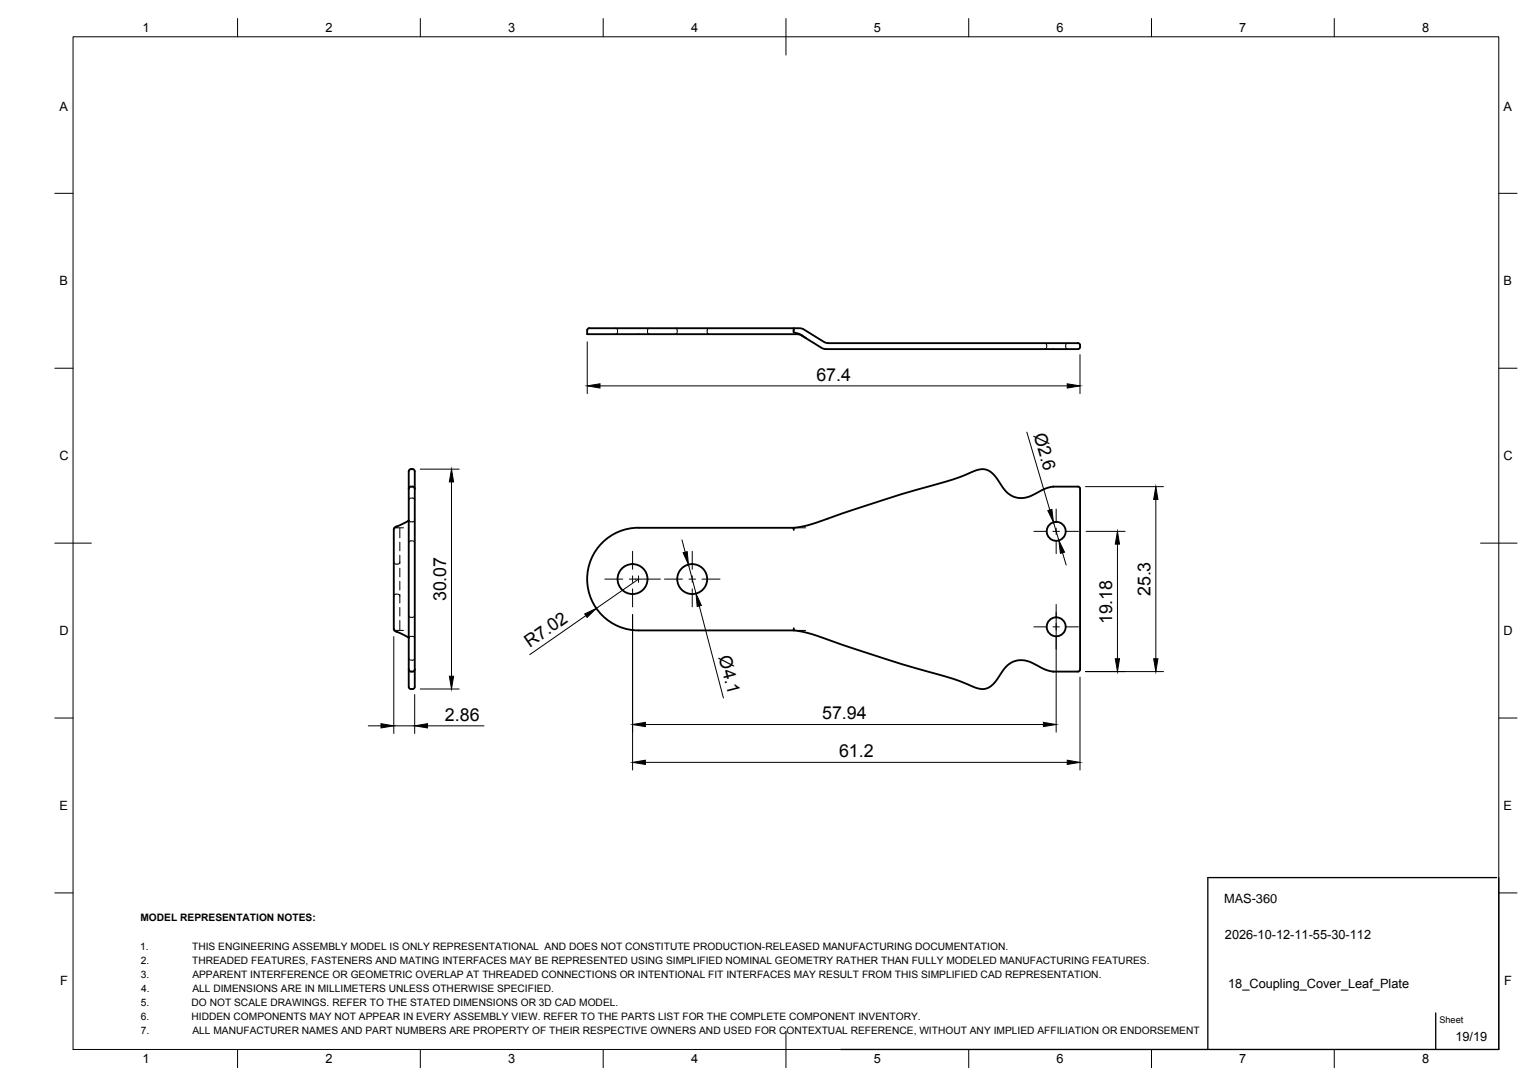
ISO-10303-21;
HEADER;
/* Generated by software containing ST-Developer
 * from STEP Tools, Inc. (www.steptools.com) 
 */

FILE_DESCRIPTION(
/* description */ (''),
/* implementation_level */ '2;1');

FILE_NAME(
/* name */ '18_Coupling_Cover_Leaf_Plate.step',
/* time_stamp */ '2026-11-04T18:53:29-08:00',
/* author */ (''),
/* organization */ (''),
/* preprocessor_version */ 'ST-DEVELOPER v20.2',
/* originating_system */ 'Autodesk Translation Framework v15.17.0.0',
/* authorisation */ '');

FILE_SCHEMA (('AUTOMOTIVE_DESIGN { 1 0 10303 214 3 1 1 }'));
ENDSEC;

DATA;
#10=MECHANICAL_DESIGN_GEOMETRIC_PRESENTATION_REPRESENTATION('',(#1336),#100031);
#217=SPHERICAL_SURFACE('',#22231,0.3);
#218=SPHERICAL_SURFACE('',#22233,0.3);
#219=SPHERICAL_SURFACE('',#22235,0.3);
#220=SPHERICAL_SURFACE('',#22237,0.3);
#221=SPHERICAL_SURFACE('',#22253,0.3);
#222=SPHERICAL_SURFACE('',#22257,0.3);
#223=SPHERICAL_SURFACE('',#22268,0.3);
#224=SPHERICAL_SURFACE('',#22270,0.3);
#1035=CIRCLE('',#22220,0.3);
#1036=CIRCLE('',#22221,0.300000000000002);
#1037=CIRCLE('',#22223,0.300000000000011);
#1038=CIRCLE('',#22224,0.3);
#1039=CIRCLE('',#22226,0.3);
#1040=CIRCLE('',#22227,0.300000000000002);
#1041=CIRCLE('',#22229,0.300000000000002);
#1042=CIRCLE('',#22230,0.3);
#1043=CIRCLE('',#22232,0.3);
#1044=CIRCLE('',#22234,0.3);
#1045=CIRCLE('',#22236,0.3);
#1046=CIRCLE('',#22238,0.3);
#1047=CIRCLE('',#22240,0.3);
#1048=CIRCLE('',#22243,0.3);
#1049=CIRCLE('',#22245,1.6);
#1050=CIRCLE('',#22246,1.6);
#1051=CIRCLE('',#22249,0.3);
#1052=CIRCLE('',#22251,0.3);
#1053=CIRCLE('',#22252,0.299999999999996);
#1054=CIRCLE('',#22254,0.299999999999999);
#1055=CIRCLE('',#22256,0.3);
#1056=CIRCLE('',#22258,0.3);
#1057=CIRCLE('',#22259,0.3);
#1058=CIRCLE('',#22260,10.3590843121497);
#1059=CIRCLE('',#22261,0.3);
#1060=CIRCLE('',#22263,1.6);
#1061=CIRCLE('',#22264,1.6);
#1062=CIRCLE('',#22266,0.3);
#1063=CIRCLE('',#22267,0.299999999999998);
#1064=CIRCLE('',#22269,0.3);
#1065=CIRCLE('',#22271,0.3);
#1066=CIRCLE('',#22272,0.3);
#1067=CIRCLE('',#22273,10.3590843136505);
#1068=CIRCLE('',#22274,0.3);
#1069=CIRCLE('',#22275,0.300000000000002);
#1070=CIRCLE('',#22276,0.300000000000001);
#1071=CIRCLE('',#22277,0.3);
#1072=CIRCLE('',#22279,0.3);
#1073=CIRCLE('',#22281,0.3);
#1074=CIRCLE('',#22282,7.0176);
#1075=CIRCLE('',#22283,6.7176);
#1076=CIRCLE('',#22285,0.3);
#1077=CIRCLE('',#22286,0.300000000000001);
#1078=CIRCLE('',#22287,0.299999999999999);
#1079=CIRCLE('',#22289,1.224);
#1080=CIRCLE('',#22292,7.0176);
#1081=CIRCLE('',#22295,1.224);
#1082=CIRCLE('',#22297,0.3);
#1083=CIRCLE('',#22298,0.299999999999999);
#1084=CIRCLE('',#22299,0.3);
#1085=CIRCLE('',#22301,0.299999999999999);
#1086=CIRCLE('',#22302,0.3);
#1087=CIRCLE('',#22303,0.3);
#1088=CIRCLE('',#22306,2.35);
#1089=CIRCLE('',#22307,2.35);
#1090=CIRCLE('',#22309,0.3);
#1091=CIRCLE('',#22310,1.3);
#1092=CIRCLE('',#22311,1.3);
#1093=CIRCLE('',#22313,1.3);
#1094=CIRCLE('',#22314,1.3);
#1095=CIRCLE('',#22316,0.3);
#1096=CIRCLE('',#22318,0.3);
#1097=CIRCLE('',#22319,2.05);
#1098=CIRCLE('',#22320,2.05);
#1099=CIRCLE('',#22322,2.05);
#1100=CIRCLE('',#22323,2.05);
#1101=CIRCLE('',#22325,2.35);
#1102=CIRCLE('',#22326,0.3);
#1103=CIRCLE('',#22328,2.35);
#1104=CIRCLE('',#22330,0.3);
#1105=CIRCLE('',#22331,1.3);
#1106=CIRCLE('',#22332,1.3);
#1107=CIRCLE('',#22334,1.3);
#1108=CIRCLE('',#22335,1.3);
#1109=CIRCLE('',#22337,0.3);
#1110=CIRCLE('',#22339,0.3);
#1111=CIRCLE('',#22340,2.05);
#1112=CIRCLE('',#22341,2.05);
#1113=CIRCLE('',#22343,2.05);
#1114=CIRCLE('',#22344,2.05);
#1115=CIRCLE('',#22346,0.3);
#1282=TOROIDAL_SURFACE('',#22280,6.7176,0.3);
#1283=TOROIDAL_SURFACE('',#22308,1.6,0.3);
#1284=TOROIDAL_SURFACE('',#22315,1.6,0.3);
#1285=TOROIDAL_SURFACE('',#22317,2.35,0.3);
#1286=TOROIDAL_SURFACE('',#22324,2.35,0.3);
#1287=TOROIDAL_SURFACE('',#22329,1.6,0.3);
#1288=TOROIDAL_SURFACE('',#22336,1.6,0.3);
#1289=TOROIDAL_SURFACE('',#22338,2.35,0.3);
#1290=TOROIDAL_SURFACE('',#22345,2.35,0.3);
#1300=SHAPE_REPRESENTATION_RELATIONSHIP('SRR','None',#100110,#1318);
#1318=ADVANCED_BREP_SHAPE_REPRESENTATION('',(#1354),#100022);
#1336=STYLED_ITEM('',(#100200),#1354);
#1354=MANIFOLD_SOLID_BREP('Body1',#20126);
#1652=PLANE('',#22241);
#1653=PLANE('',#22244);
#1654=PLANE('',#22247);
#1655=PLANE('',#22262);
#1656=PLANE('',#22288);
#1657=PLANE('',#22293);
#1658=PLANE('',#22296);
#1659=PLANE('',#22305);
#1660=PLANE('',#22327);
#1661=PLANE('',#22347);
#1662=PLANE('',#22350);
#1782=FACE_BOUND('',#7296,.T.);
#1783=FACE_BOUND('',#7297,.T.);
#1784=FACE_BOUND('',#7308,.T.);
#1785=FACE_BOUND('',#7309,.T.);
#1786=FACE_BOUND('',#7342,.T.);
#1787=FACE_BOUND('',#7343,.T.);
#1788=FACE_BOUND('',#7351,.T.);
#1789=FACE_BOUND('',#7352,.T.);
#1978=ELLIPSE('',#22290,2.28040158611643,0.428995210802967);
#1979=ELLIPSE('',#22294,2.23144347816224,0.415540935948683);
#3183=LINE('',#97807,#4470);
#3184=LINE('',#97810,#4471);
#3185=LINE('',#97816,#4472);
#3186=LINE('',#97818,#4473);
#3187=LINE('',#97823,#4474);
#3188=LINE('',#97826,#4475);
#3189=LINE('',#97831,#4476);
#3190=LINE('',#97833,#4477);
#3191=LINE('',#97844,#4478);
#3192=LINE('',#97847,#4479);
#3193=LINE('',#97850,#4480);
#3194=LINE('',#97851,#4481);
#3195=LINE('',#97854,#4482);
#3196=LINE('',#97858,#4483);
#3197=LINE('',#97889,#4484);
#3198=LINE('',#97923,#4485);
#3199=LINE('',#97929,#4486);
#3200=LINE('',#97932,#4487);
#3201=LINE('',#97937,#4488);
#3202=LINE('',#97939,#4489);
#3203=LINE('',#98313,#4490);
#3204=LINE('',#98546,#4491);
#3205=LINE('',#98555,#4492);
#3206=LINE('',#98952,#4493);
#3207=LINE('',#99248,#4494);
#3208=LINE('',#99251,#4495);
#3209=LINE('',#99259,#4496);
#3210=LINE('',#99261,#4497);
#3211=LINE('',#99394,#4498);
#3212=LINE('',#99396,#4499);
#3213=LINE('',#99400,#4500);
#3214=LINE('',#99426,#4501);
#3215=LINE('',#99452,#4502);
#3216=LINE('',#99455,#4503);
#3217=LINE('',#99551,#4504);
#3218=LINE('',#99636,#4505);
#3219=LINE('',#99637,#4506);
#3220=LINE('',#99651,#4507);
#3221=LINE('',#99665,#4508);
#3222=LINE('',#99674,#4509);
#3223=LINE('',#99685,#4510);
#3224=LINE('',#99699,#4511);
#3225=LINE('',#99707,#4512);
#3226=LINE('',#99709,#4513);
#4470=VECTOR('',#27502,10.);
#4471=VECTOR('',#27505,10.);
#4472=VECTOR('',#27510,10.);
#4473=VECTOR('',#27513,10.);
#4474=VECTOR('',#27518,10.);
#4475=VECTOR('',#27521,10.);
#4476=VECTOR('',#27526,10.);
#4477=VECTOR('',#27529,10.);
#4478=VECTOR('',#27548,10.);
#4479=VECTOR('',#27551,10.);
#4480=VECTOR('',#27554,10.);
#4481=VECTOR('',#27555,10.);
#4482=VECTOR('',#27558,10.);
#4483=VECTOR('',#27563,10.);
#4484=VECTOR('',#27564,10.);
#4485=VECTOR('',#27573,10.);
#4486=VECTOR('',#27580,10.);
#4487=VECTOR('',#27583,10.);
#4488=VECTOR('',#27590,10.);
#4489=VECTOR('',#27593,10.);
#4490=VECTOR('',#27602,10.);
#4491=VECTOR('',#27607,10.);
#4492=VECTOR('',#27616,10.);
#4493=VECTOR('',#27629,10.);
#4494=VECTOR('',#27642,10.);
#4495=VECTOR('',#27645,10.);
#4496=VECTOR('',#27656,10.);
#4497=VECTOR('',#27657,10.);
#4498=VECTOR('',#27666,10.);
#4499=VECTOR('',#27667,10.);
#4500=VECTOR('',#27670,10.);
#4501=VECTOR('',#27675,10.);
#4502=VECTOR('',#27682,10.);
#4503=VECTOR('',#27685,10.);
#4504=VECTOR('',#27696,10.);
#4505=VECTOR('',#27705,10.);
#4506=VECTOR('',#27706,10.);
#4507=VECTOR('',#27723,1.3);
#4508=VECTOR('',#27742,2.05);
#4509=VECTOR('',#27755,10.);
#4510=VECTOR('',#27768,1.3);
#4511=VECTOR('',#27787,2.05);
#4512=VECTOR('',#27800,10.);
#4513=VECTOR('',#27803,10.);
#4980=CYLINDRICAL_SURFACE('',#22219,0.3);
#4981=CYLINDRICAL_SURFACE('',#22222,0.3);
#4982=CYLINDRICAL_SURFACE('',#22225,0.3);
#4983=CYLINDRICAL_SURFACE('',#22228,0.3);
#4984=CYLINDRICAL_SURFACE('',#22239,0.3);
#4985=CYLINDRICAL_SURFACE('',#22242,0.3);
#4986=CYLINDRICAL_SURFACE('',#22248,0.3);
#4987=CYLINDRICAL_SURFACE('',#22250,0.300092189998616);
#4988=CYLINDRICAL_SURFACE('',#22255,0.3);
#4989=CYLINDRICAL_SURFACE('',#22265,0.300092189989763);
#4990=CYLINDRICAL_SURFACE('',#22278,0.3);
#4991=CYLINDRICAL_SURFACE('',#22284,0.3);
#4992=CYLINDRICAL_SURFACE('',#22291,7.0176);
#4993=CYLINDRICAL_SURFACE('',#22300,1.224);
#4994=CYLINDRICAL_SURFACE('',#22304,1.224);
#4995=CYLINDRICAL_SURFACE('',#22312,1.3);
#4996=CYLINDRICAL_SURFACE('',#22321,2.05);
#4997=CYLINDRICAL_SURFACE('',#22333,1.3);
#4998=CYLINDRICAL_SURFACE('',#22342,2.05);
#4999=CYLINDRICAL_SURFACE('',#22348,1.224);
#5000=CYLINDRICAL_SURFACE('',#22349,1.224);
#6039=FACE_OUTER_BOUND('',#7284,.T.);
#6040=FACE_OUTER_BOUND('',#7285,.T.);
#6041=FACE_OUTER_BOUND('',#7286,.T.);
#6042=FACE_OUTER_BOUND('',#7287,.T.);
#6043=FACE_OUTER_BOUND('',#7288,.T.);
#6044=FACE_OUTER_BOUND('',#7289,.T.);
#6045=FACE_OUTER_BOUND('',#7290,.T.);
#6046=FACE_OUTER_BOUND('',#7291,.T.);
#6047=FACE_OUTER_BOUND('',#7292,.T.);
#6048=FACE_OUTER_BOUND('',#7293,.T.);
#6049=FACE_OUTER_BOUND('',#7294,.T.);
#6050=FACE_OUTER_BOUND('',#7295,.T.);
#6051=FACE_OUTER_BOUND('',#7298,.T.);
#6052=FACE_OUTER_BOUND('',#7299,.T.);
#6053=FACE_OUTER_BOUND('',#7300,.T.);
#6054=FACE_OUTER_BOUND('',#7301,.T.);
#6055=FACE_OUTER_BOUND('',#7302,.T.);
#6056=FACE_OUTER_BOUND('',#7303,.T.);
#6057=FACE_OUTER_BOUND('',#7304,.T.);
#6058=FACE_OUTER_BOUND('',#7305,.T.);
#6059=FACE_OUTER_BOUND('',#7306,.T.);
#6060=FACE_OUTER_BOUND('',#7307,.T.);
#6061=FACE_OUTER_BOUND('',#7310,.T.);
#6062=FACE_OUTER_BOUND('',#7311,.T.);
#6063=FACE_OUTER_BOUND('',#7312,.T.);
#6064=FACE_OUTER_BOUND('',#7313,.T.);
#6065=FACE_OUTER_BOUND('',#7314,.T.);
#6066=FACE_OUTER_BOUND('',#7315,.T.);
#6067=FACE_OUTER_BOUND('',#7316,.T.);
#6068=FACE_OUTER_BOUND('',#7317,.T.);
#6069=FACE_OUTER_BOUND('',#7318,.T.);
#6070=FACE_OUTER_BOUND('',#7319,.T.);
#6071=FACE_OUTER_BOUND('',#7320,.T.);
#6072=FACE_OUTER_BOUND('',#7321,.T.);
#6073=FACE_OUTER_BOUND('',#7322,.T.);
#6074=FACE_OUTER_BOUND('',#7323,.T.);
#6075=FACE_OUTER_BOUND('',#7324,.T.);
#6076=FACE_OUTER_BOUND('',#7325,.T.);
#6077=FACE_OUTER_BOUND('',#7326,.T.);
#6078=FACE_OUTER_BOUND('',#7327,.T.);
#6079=FACE_OUTER_BOUND('',#7328,.T.);
#6080=FACE_OUTER_BOUND('',#7329,.T.);
#6081=FACE_OUTER_BOUND('',#7330,.T.);
#6082=FACE_OUTER_BOUND('',#7331,.T.);
#6083=FACE_OUTER_BOUND('',#7332,.T.);
#6084=FACE_OUTER_BOUND('',#7333,.T.);
#6085=FACE_OUTER_BOUND('',#7334,.T.);
#6086=FACE_OUTER_BOUND('',#7335,.T.);
#6087=FACE_OUTER_BOUND('',#7336,.T.);
#6088=FACE_OUTER_BOUND('',#7337,.T.);
#6089=FACE_OUTER_BOUND('',#7338,.T.);
#6090=FACE_OUTER_BOUND('',#7339,.T.);
#6091=FACE_OUTER_BOUND('',#7340,.T.);
#6092=FACE_OUTER_BOUND('',#7341,.T.);
#6093=FACE_OUTER_BOUND('',#7344,.T.);
#6094=FACE_OUTER_BOUND('',#7345,.T.);
#6095=FACE_OUTER_BOUND('',#7346,.T.);
#6096=FACE_OUTER_BOUND('',#7347,.T.);
#6097=FACE_OUTER_BOUND('',#7348,.T.);
#6098=FACE_OUTER_BOUND('',#7349,.T.);
#6099=FACE_OUTER_BOUND('',#7350,.T.);
#6100=FACE_OUTER_BOUND('',#7353,.T.);
#6101=FACE_OUTER_BOUND('',#7354,.T.);
#6102=FACE_OUTER_BOUND('',#7355,.T.);
#6103=FACE_OUTER_BOUND('',#7356,.T.);
#6104=FACE_OUTER_BOUND('',#7357,.T.);
#6105=FACE_OUTER_BOUND('',#7358,.T.);
#6106=FACE_OUTER_BOUND('',#7359,.T.);
#6107=FACE_OUTER_BOUND('',#7360,.T.);
#6108=FACE_OUTER_BOUND('',#7361,.T.);
#6109=FACE_OUTER_BOUND('',#7362,.T.);
#7284=EDGE_LOOP('',(#18301,#18302,#18303,#18304));
#7285=EDGE_LOOP('',(#18305,#18306,#18307,#18308));
#7286=EDGE_LOOP('',(#18309,#18310,#18311,#18312));
#7287=EDGE_LOOP('',(#18313,#18314,#18315,#18316));
#7288=EDGE_LOOP('',(#18317,#18318,#18319));
#7289=EDGE_LOOP('',(#18320,#18321,#18322));
#7290=EDGE_LOOP('',(#18323,#18324,#18325));
#7291=EDGE_LOOP('',(#18326,#18327,#18328));
#7292=EDGE_LOOP('',(#18329,#18330,#18331,#18332));
#7293=EDGE_LOOP('',(#18333,#18334,#18335,#18336));
#7294=EDGE_LOOP('',(#18337,#18338,#18339,#18340));
#7295=EDGE_LOOP('',(#18341,#18342,#18343,#18344,#18345,#18346));
#7296=EDGE_LOOP('',(#18347));
#7297=EDGE_LOOP('',(#18348));
#7298=EDGE_LOOP('',(#18349,#18350,#18351,#18352));
#7299=EDGE_LOOP('',(#18353,#18354,#18355,#18356));
#7300=EDGE_LOOP('',(#18357,#18358,#18359,#18360));
#7301=EDGE_LOOP('',(#18361,#18362,#18363));
#7302=EDGE_LOOP('',(#18364,#18365,#18366,#18367));
#7303=EDGE_LOOP('',(#18368,#18369,#18370));
#7304=EDGE_LOOP('',(#18371,#18372,#18373,#18374));
#7305=EDGE_LOOP('',(#18375,#18376,#18377,#18378,#18379,#18380,#18381,#18382,
#18383,#18384,#18385,#18386));
#7306=EDGE_LOOP('',(#18387,#18388,#18389,#18390));
#7307=EDGE_LOOP('',(#18391,#18392,#18393,#18394,#18395,#18396));
#7308=EDGE_LOOP('',(#18397));
#7309=EDGE_LOOP('',(#18398));
#7310=EDGE_LOOP('',(#18399,#18400,#18401,#18402));
#7311=EDGE_LOOP('',(#18403,#18404,#18405));
#7312=EDGE_LOOP('',(#18406,#18407,#18408));
#7313=EDGE_LOOP('',(#18409,#18410,#18411,#18412));
#7314=EDGE_LOOP('',(#18413,#18414,#18415,#18416,#18417,#18418,#18419,#18420,
#18421,#18422,#18423,#18424));
#7315=EDGE_LOOP('',(#18425,#18426,#18427,#18428));
#7316=EDGE_LOOP('',(#18429,#18430,#18431,#18432));
#7317=EDGE_LOOP('',(#18433,#18434,#18435,#18436));
#7318=EDGE_LOOP('',(#18437,#18438,#18439,#18440));
#7319=EDGE_LOOP('',(#18441,#18442,#18443,#18444));
#7320=EDGE_LOOP('',(#18445,#18446,#18447,#18448));
#7321=EDGE_LOOP('',(#18449,#18450,#18451,#18452));
#7322=EDGE_LOOP('',(#18453,#18454,#18455,#18456));
#7323=EDGE_LOOP('',(#18457,#18458,#18459,#18460));
#7324=EDGE_LOOP('',(#18461,#18462,#18463,#18464));
#7325=EDGE_LOOP('',(#18465,#18466,#18467,#18468));
#7326=EDGE_LOOP('',(#18469,#18470,#18471,#18472));
#7327=EDGE_LOOP('',(#18473,#18474,#18475,#18476,#18477,#18478,#18479,#18480,
#18481));
#7328=EDGE_LOOP('',(#18482,#18483,#18484,#18485));
#7329=EDGE_LOOP('',(#18486,#18487,#18488,#18489,#18490,#18491,#18492,#18493,
#18494));
#7330=EDGE_LOOP('',(#18495,#18496,#18497,#18498));
#7331=EDGE_LOOP('',(#18499,#18500,#18501,#18502,#18503));
#7332=EDGE_LOOP('',(#18504,#18505,#18506,#18507));
#7333=EDGE_LOOP('',(#18508,#18509,#18510));
#7334=EDGE_LOOP('',(#18511,#18512,#18513,#18514));
#7335=EDGE_LOOP('',(#18515,#18516,#18517,#18518));
#7336=EDGE_LOOP('',(#18519,#18520,#18521,#18522,#18523));
#7337=EDGE_LOOP('',(#18524,#18525,#18526,#18527));
#7338=EDGE_LOOP('',(#18528,#18529,#18530,#18531));
#7339=EDGE_LOOP('',(#18532,#18533,#18534));
#7340=EDGE_LOOP('',(#18535,#18536,#18537,#18538));
#7341=EDGE_LOOP('',(#18539,#18540,#18541,#18542));
#7342=EDGE_LOOP('',(#18543));
#7343=EDGE_LOOP('',(#18544));
#7344=EDGE_LOOP('',(#18545,#18546,#18547,#18548,#18549));
#7345=EDGE_LOOP('',(#18550,#18551,#18552,#18553,#18554,#18555));
#7346=EDGE_LOOP('',(#18556,#18557,#18558,#18559,#18560));
#7347=EDGE_LOOP('',(#18561,#18562,#18563,#18564,#18565));
#7348=EDGE_LOOP('',(#18566,#18567,#18568,#18569,#18570,#18571));
#7349=EDGE_LOOP('',(#18572,#18573,#18574,#18575,#18576));
#7350=EDGE_LOOP('',(#18577,#18578,#18579,#18580,#18581,#18582));
#7351=EDGE_LOOP('',(#18583));
#7352=EDGE_LOOP('',(#18584));
#7353=EDGE_LOOP('',(#18585,#18586,#18587,#18588,#18589));
#7354=EDGE_LOOP('',(#18590,#18591,#18592,#18593,#18594,#18595));
#7355=EDGE_LOOP('',(#18596,#18597,#18598,#18599,#18600));
#7356=EDGE_LOOP('',(#18601,#18602,#18603,#18604,#18605));
#7357=EDGE_LOOP('',(#18606,#18607,#18608,#18609,#18610,#18611));
#7358=EDGE_LOOP('',(#18612,#18613,#18614,#18615,#18616));
#7359=EDGE_LOOP('',(#18617,#18618,#18619,#18620,#18621,#18622));
#7360=EDGE_LOOP('',(#18623,#18624,#18625,#18626));
#7361=EDGE_LOOP('',(#18627,#18628,#18629,#18630));
#7362=EDGE_LOOP('',(#18631,#18632,#18633,#18634));
#8003=B_SPLINE_CURVE_WITH_KNOTS('',3,(#97860,#97861,#97862,#97863,#97864,
#97865,#97866,#97867,#97868,#97869,#97870,#97871,#97872,#97873,#97874,#97875,
#97876,#97877,#97878,#97879,#97880,#97881,#97882,#97883,#97884,#97885,#97886,
#97887),.UNSPECIFIED.,.F.,.F.,(4,1,1,1,1,1,1,1,1,1,1,1,1,1,1,1,1,1,1,1,
1,1,1,1,1,4),(3.41679525229117E-14,0.241483590676928,0.482967181353822,
0.96593436270761,1.2074179533845,1.4489015440614,1.69038513473829,1.81112693007674,
1.87149782774596,1.90168327658057,1.93186872541519,2.05261052075363,2.11298141842286,
2.17335231609208,2.2337232137613,2.29409411143053,2.35446500909975,2.41483590676897,
2.53557770210742,2.65631949744587,2.77706129278432,2.89780308812276,3.01854488346121,
3.13928667879966,3.2600284741381,3.38077026947655),.UNSPECIFIED.);
#8004=B_SPLINE_CURVE_WITH_KNOTS('',3,(#97890,#97891,#97892,#97893,#97894,
#97895,#97896,#97897,#97898,#97899,#97900,#97901,#97902,#97903,#97904,#97905,
#97906,#97907,#97908,#97909,#97910,#97911,#97912,#97913,#97914,#97915),
 .UNSPECIFIED.,.F.,.F.,(4,1,1,1,1,1,1,1,1,1,1,1,1,1,1,1,1,1,1,1,1,1,1,4),
(0.00128110943246098,0.1220229047709,0.242764700109339,0.363506495447778,
0.484248290786216,0.604990086124655,0.725731881463094,0.846473676801533,
0.906844574470752,0.967215472139972,1.02758636980919,1.08795726747841,1.14832816514763,
1.20869906281685,1.26906996048607,1.32944085815529,1.45018265349373,1.6916662441706,
1.93314983484748,2.17463342552436,2.41611701620124,2.89908419755499,3.14056778823187,
3.38205137890875),.UNSPECIFIED.);
#8005=B_SPLINE_CURVE_WITH_KNOTS('',3,(#98083,#98084,#98085,#98086,#98087,
#98088,#98089,#98090,#98091,#98092,#98093,#98094,#98095,#98096,#98097,#98098,
#98099,#98100,#98101,#98102,#98103,#98104,#98105,#98106,#98107,#98108,#98109,
#98110),.UNSPECIFIED.,.F.,.F.,(4,1,1,1,1,1,1,1,1,1,1,1,1,1,1,1,1,1,1,1,
1,1,1,1,1,4),(-3.38077026947655,-3.2600284741381,-3.13928667879966,-3.01854488346121,
-2.89780308812276,-2.77706129278432,-2.65631949744587,-2.53557770210742,
-2.41483590676897,-2.35446500909975,-2.29409411143053,-2.2337232137613,
-2.17335231609208,-2.11298141842286,-2.05261052075363,-1.93186872541519,
-1.90168327658057,-1.87149782774596,-1.81112693007674,-1.69038513473829,
-1.4489015440614,-1.2074179533845,-0.96593436270761,-0.482967181353822,
-0.241483590676928,-3.41679525229117E-14),.UNSPECIFIED.);
#8006=B_SPLINE_CURVE_WITH_KNOTS('',3,(#98253,#98254,#98255,#98256,#98257,
#98258,#98259,#98260,#98261,#98262,#98263,#98264,#98265,#98266,#98267,#98268,
#98269,#98270,#98271,#98272,#98273,#98274,#98275,#98276,#98277,#98278,#98279),
 .UNSPECIFIED.,.F.,.F.,(4,1,1,1,1,1,1,1,1,1,1,1,1,1,1,1,1,1,1,1,1,1,1,1,
4),(-3.41890546063757,-3.17478943294163,-2.93067340524569,-2.4424413498538,
-2.19832532215786,-1.95420929446192,-1.83215128061395,-1.71009326676598,
-1.46597723907004,-1.34391922522207,-1.2218612113741,-1.1913467079121,-1.16083220445011,
-1.09980319752612,-1.03877419060214,-0.977745183678154,-0.855687169830184,
-0.733629155982213,-0.611571142134242,-0.489513128286272,-0.367455114438301,
-0.24539710059033,-0.12333908674236,-0.0623100798183742,-0.00128107289438891),
 .UNSPECIFIED.);
#8007=B_SPLINE_CURVE_WITH_KNOTS('',3,(#98281,#98282,#98283,#98284,#98285,
#98286,#98287,#98288,#98289,#98290),.UNSPECIFIED.,.F.,.F.,(4,3,3,4),(0.,
0.0193508010140011,0.0377654905305143,0.0545713498196275),.UNSPECIFIED.);
#8008=B_SPLINE_CURVE_WITH_KNOTS('',3,(#98292,#98293,#98294,#98295),
 .UNSPECIFIED.,.F.,.F.,(4,4),(-0.324683822128034,0.),.UNSPECIFIED.);
#8009=B_SPLINE_CURVE_WITH_KNOTS('',3,(#98297,#98298,#98299,#98300,#98301,
#98302,#98303,#98304,#98305,#98306,#98307,#98308,#98309),.UNSPECIFIED.,
 .F.,.F.,(4,3,3,3,4),(0.,0.0219603143385993,0.0442891506855458,0.067805646823492,
0.0861862379095711),.UNSPECIFIED.);
#8010=B_SPLINE_CURVE_WITH_KNOTS('',3,(#98315,#98316,#98317,#98318),
 .UNSPECIFIED.,.F.,.F.,(4,4),(-0.0771338280522776,-3.23236617932421E-6),
 .UNSPECIFIED.);
#8011=B_SPLINE_CURVE_WITH_KNOTS('',3,(#98320,#98321,#98322,#98323),
 .UNSPECIFIED.,.F.,.F.,(4,4),(0.,0.0523726503223924),.UNSPECIFIED.);
#8012=B_SPLINE_CURVE_WITH_KNOTS('',3,(#98325,#98326,#98327,#98328,#98329,
#98330,#98331,#98332,#98333,#98334,#98335,#98336,#98337,#98338,#98339,#98340,
#98341,#98342,#98343,#98344,#98345,#98346),.UNSPECIFIED.,.F.,.F.,(4,3,3,
3,3,3,3,4),(-0.324714104720811,-0.275894006039472,-0.219811108021725,-0.164858331016294,
-0.117285452027523,-0.0705633041497707,-0.0225934601586412,-2.03395786214367E-15),
 .UNSPECIFIED.);
#8013=B_SPLINE_CURVE_WITH_KNOTS('',3,(#98347,#98348,#98349,#98350),
 .UNSPECIFIED.,.F.,.F.,(4,4),(0.,0.0900393973869889),.UNSPECIFIED.);
#8014=B_SPLINE_CURVE_WITH_KNOTS('',3,(#98487,#98488,#98489,#98490,#98491,
#98492,#98493,#98494,#98495,#98496,#98497,#98498,#98499,#98500,#98501,#98502,
#98503,#98504,#98505,#98506,#98507,#98508,#98509,#98510,#98511,#98512,#98513),
 .UNSPECIFIED.,.F.,.F.,(4,1,1,1,1,1,1,1,1,1,1,1,1,1,1,1,1,1,1,1,1,1,1,1,
4),(0.00128107289438891,0.0623100798183742,0.12333908674236,0.24539710059033,
0.367455114438301,0.489513128286272,0.611571142134242,0.733629155982213,
0.855687169830184,0.977745183678154,1.03877419060214,1.09980319752612,1.16083220445011,
1.1913467079121,1.2218612113741,1.34391922522207,1.46597723907004,1.71009326676598,
1.83215128061395,1.95420929446192,2.19832532215786,2.4424413498538,2.93067340524569,
3.17478943294163,3.41890546063757),.UNSPECIFIED.);
#8015=B_SPLINE_CURVE_WITH_KNOTS('',3,(#98517,#98518,#98519,#98520,#98521,
#98522,#98523,#98524,#98525,#98526,#98527,#98528,#98529,#98530,#98531,#98532,
#98533,#98534,#98535,#98536,#98537,#98538,#98539,#98540,#98541,#98542,#98543,
#98544,#98545),.UNSPECIFIED.,.F.,.F.,(4,1,1,1,1,1,1,1,1,1,1,1,1,1,1,1,1,
1,1,1,1,1,1,1,1,1,4),(0.,0.244116027696041,0.488232055392083,0.976464110784166,
1.22058013848021,1.46469616617625,1.70881219387229,1.83087020772031,1.89189921464432,
1.95292822156833,2.07498623541635,2.13601524234036,2.19704424926437,2.25807325618838,
2.28858775965039,2.31910226311239,2.3801312700364,2.44116027696041,2.56321829080843,
2.68527630465646,2.80733431850448,2.9293923323525,3.05145034620052,3.17350836004854,
3.29556637389656,3.35659538082057,3.41762438774458),.UNSPECIFIED.);
#8016=B_SPLINE_CURVE_WITH_KNOTS('',3,(#98707,#98708,#98709,#98710,#98711,
#98712,#98713,#98714,#98715,#98716,#98717,#98718,#98719,#98720,#98721,#98722,
#98723,#98724,#98725,#98726,#98727,#98728,#98729,#98730,#98731,#98732,#98733,
#98734,#98735),.UNSPECIFIED.,.F.,.F.,(4,1,1,1,1,1,1,1,1,1,1,1,1,1,1,1,1,
1,1,1,1,1,1,1,1,1,4),(-3.41762438774458,-3.35659538082057,-3.29556637389656,
-3.17350836004854,-3.05145034620052,-2.9293923323525,-2.80733431850448,
-2.68527630465646,-2.56321829080843,-2.44116027696041,-2.3801312700364,
-2.31910226311239,-2.28858775965039,-2.25807325618838,-2.19704424926437,
-2.13601524234036,-2.07498623541635,-1.95292822156833,-1.89189921464432,
-1.83087020772031,-1.70881219387229,-1.46469616617625,-1.22058013848021,
-0.976464110784166,-0.488232055392083,-0.244116027696041,0.),
 .UNSPECIFIED.);
#8017=B_SPLINE_CURVE_WITH_KNOTS('',3,(#98878,#98879,#98880,#98881,#98882,
#98883,#98884,#98885,#98886,#98887,#98888,#98889,#98890,#98891,#98892,#98893,
#98894,#98895,#98896,#98897,#98898,#98899,#98900,#98901,#98902,#98903),
 .UNSPECIFIED.,.F.,.F.,(4,1,1,1,1,1,1,1,1,1,1,1,1,1,1,1,1,1,1,1,1,1,1,4),
(-3.38205137890875,-3.14056778823187,-2.89908419755499,-2.41611701620124,
-2.17463342552436,-1.93314983484748,-1.6916662441706,-1.45018265349373,
-1.32944085815529,-1.26906996048607,-1.20869906281685,-1.14832816514763,
-1.08795726747841,-1.02758636980919,-0.967215472139972,-0.906844574470752,
-0.846473676801533,-0.725731881463094,-0.604990086124655,-0.484248290786216,
-0.363506495447778,-0.242764700109339,-0.1220229047709,-0.00128110943246098),
 .UNSPECIFIED.);
#8018=B_SPLINE_CURVE_WITH_KNOTS('',3,(#98905,#98906,#98907,#98908),
 .UNSPECIFIED.,.F.,.F.,(4,4),(0.,0.0900415523927057),.UNSPECIFIED.);
#8019=B_SPLINE_CURVE_WITH_KNOTS('',3,(#98910,#98911,#98912,#98913,#98914,
#98915,#98916,#98917,#98918,#98919,#98920,#98921,#98922,#98923,#98924,#98925,
#98926,#98927,#98928,#98929,#98930,#98931),.UNSPECIFIED.,.F.,.F.,(4,3,3,
3,3,3,3,4),(-0.324714104720872,-0.276900417543011,-0.230088047477266,-0.182596766871424,
-0.130785402885425,-0.0701896017717822,-0.0219763511414979,-9.48740063601895E-16),
 .UNSPECIFIED.);
#8020=B_SPLINE_CURVE_WITH_KNOTS('',3,(#98933,#98934,#98935,#98936),
 .UNSPECIFIED.,.F.,.F.,(4,4),(0.,0.0523713743724485),.UNSPECIFIED.);
#8021=B_SPLINE_CURVE_WITH_KNOTS('',3,(#98938,#98939,#98940,#98941,#98942,
#98943,#98944,#98945,#98946,#98947,#98948,#98949,#98950),.UNSPECIFIED.,
 .F.,.F.,(4,3,3,3,4),(-0.0771330433688407,-0.0532273517721988,-0.0290520233522164,
-0.00468787888284027,-1.22307313571325E-14),.UNSPECIFIED.);
#8022=B_SPLINE_CURVE_WITH_KNOTS('',3,(#98956,#98957,#98958,#98959,#98960,
#98961,#98962,#98963,#98964,#98965,#98966,#98967,#98968),.UNSPECIFIED.,
 .F.,.F.,(4,3,3,3,4),(1.94736699620138E-16,0.0234829329857791,0.0461120293622291,
0.068043235237682,0.0861862379095512),.UNSPECIFIED.);
#8023=B_SPLINE_CURVE_WITH_KNOTS('',3,(#98970,#98971,#98972,#98973),
 .UNSPECIFIED.,.F.,.F.,(4,4),(-0.324683822128098,0.),.UNSPECIFIED.);
#8024=B_SPLINE_CURVE_WITH_KNOTS('',3,(#98974,#98975,#98976,#98977,#98978,
#98979,#98980,#98981,#98982,#98983),.UNSPECIFIED.,.F.,.F.,(4,3,3,4),(0.,
0.0183070922409377,0.0374313150775962,0.0545713498196216),.UNSPECIFIED.);
#8025=B_SPLINE_CURVE_WITH_KNOTS('',3,(#99136,#99137,#99138,#99139),
 .UNSPECIFIED.,.F.,.F.,(4,4),(-0.0900415523927057,0.),.UNSPECIFIED.);
#8026=B_SPLINE_CURVE_WITH_KNOTS('',3,(#99163,#99164,#99165,#99166),
 .UNSPECIFIED.,.F.,.F.,(4,4),(9.48740063601895E-16,0.324714104720872),
 .UNSPECIFIED.);
#8027=B_SPLINE_CURVE_WITH_KNOTS('',3,(#99188,#99189,#99190,#99191),
 .UNSPECIFIED.,.F.,.F.,(4,4),(-0.0523713743724485,0.),.UNSPECIFIED.);
#8028=B_SPLINE_CURVE_WITH_KNOTS('',3,(#99224,#99225,#99226,#99227,#99228,
#99229),.UNSPECIFIED.,.F.,.F.,(4,2,4),(1.22307313571325E-14,0.0771338280521436,
0.0784358874721452),.UNSPECIFIED.);
#8029=B_SPLINE_CURVE_WITH_KNOTS('',3,(#99230,#99231,#99232,#99233,#99234,
#99235,#99236,#99237,#99238,#99239,#99240,#99241,#99242,#99243,#99244,#99245),
 .UNSPECIFIED.,.F.,.F.,(4,2,2,2,2,2,2,4),(-0.00022668224436296,0.,0.00761586611745941,
0.0150248302469871,0.0236797709907964,0.0310979044849912,0.0368289860988756,
0.0428654183141884),.UNSPECIFIED.);
#8030=B_SPLINE_CURVE_WITH_KNOTS('',3,(#99262,#99263,#99264,#99265,#99266,
#99267,#99268,#99269,#99270,#99271,#99272,#99273,#99274,#99275,#99276,#99277),
 .UNSPECIFIED.,.F.,.F.,(4,2,2,2,2,2,2,4),(-0.0509737628840132,-0.0507050440328071,
-0.0417234339127921,-0.0329872447452147,-0.0226497365660009,-0.0138121252681416,
-0.00708364657956319,0.),.UNSPECIFIED.);
#8031=B_SPLINE_CURVE_WITH_KNOTS('',3,(#99301,#99302,#99303,#99304),
 .UNSPECIFIED.,.F.,.F.,(4,4),(-0.0523726503223924,0.),.UNSPECIFIED.);
#8032=B_SPLINE_CURVE_WITH_KNOTS('',3,(#99336,#99337,#99338,#99339,#99340,
#99341),.UNSPECIFIED.,.F.,.F.,(4,2,4),(-0.00130205941990691,0.,0.0771338280522776),
 .UNSPECIFIED.);
#8033=B_SPLINE_CURVE_WITH_KNOTS('',3,(#99364,#99365,#99366,#99367),
 .UNSPECIFIED.,.F.,.F.,(4,4),(2.03395786214367E-15,0.324714104720811),
 .UNSPECIFIED.);
#8034=B_SPLINE_CURVE_WITH_KNOTS('',3,(#99388,#99389,#99390,#99391),
 .UNSPECIFIED.,.F.,.F.,(4,4),(-0.0900393973869889,0.),.UNSPECIFIED.);
#8035=B_SPLINE_CURVE_WITH_KNOTS('',3,(#99404,#99405,#99406,#99407,#99408,
#99409),.UNSPECIFIED.,.F.,.F.,(4,2,4),(-0.0750162613442511,-0.0337302597397184,
-6.17748433559551E-7),.UNSPECIFIED.);
#8036=B_SPLINE_CURVE_WITH_KNOTS('',3,(#99410,#99411,#99412,#99413,#99414,
#99415,#99416,#99417,#99418,#99419,#99420,#99421,#99422,#99423),
 .UNSPECIFIED.,.F.,.F.,(4,2,2,2,2,2,4),(-0.0264541140821501,-0.017390110288006,
-0.011146376492299,-0.00376454098685937,-0.00160326722853797,-0.00077940018444644,
0.),.UNSPECIFIED.);
#8037=B_SPLINE_CURVE_WITH_KNOTS('',3,(#99430,#99431,#99432,#99433,#99434,
#99435,#99436,#99437,#99438,#99439,#99440,#99441),.UNSPECIFIED.,.F.,.F.,
(4,2,2,2,2,4),(-0.0641362373983827,-0.0612026902636628,-0.0580728061365246,
-0.0499071281293661,-0.0252640899793066,-5.18312203295901E-7),
 .UNSPECIFIED.);
#8038=B_SPLINE_CURVE_WITH_KNOTS('',3,(#99443,#99444,#99445,#99446,#99447,
#99448),.UNSPECIFIED.,.F.,.F.,(4,2,4),(-0.0743753002286862,-0.0371638184856682,
-1.00312867462312E-6),.UNSPECIFIED.);
#8039=B_SPLINE_CURVE_WITH_KNOTS('',3,(#99480,#99481,#99482,#99483),
 .UNSPECIFIED.,.F.,.F.,(4,4),(0.,0.261923043407585),.UNSPECIFIED.);
#8040=B_SPLINE_CURVE_WITH_KNOTS('',3,(#99541,#99542,#99543,#99544),
 .UNSPECIFIED.,.F.,.F.,(4,4),(-0.0545713498196275,0.),.UNSPECIFIED.);
#8041=B_SPLINE_CURVE_WITH_KNOTS('',3,(#99547,#99548,#99549,#99550),
 .UNSPECIFIED.,.F.,.F.,(4,4),(-0.0545713498196216,0.),.UNSPECIFIED.);
#8042=B_SPLINE_CURVE_WITH_KNOTS('',3,(#99572,#99573,#99574,#99575),
 .UNSPECIFIED.,.F.,.F.,(4,4),(0.0627607787207755,0.324683822128098),
 .UNSPECIFIED.);
#9759=VERTEX_POINT('',#97803);
#9760=VERTEX_POINT('',#97804);
#9761=VERTEX_POINT('',#97806);
#9762=VERTEX_POINT('',#97808);
#9763=VERTEX_POINT('',#97812);
#9764=VERTEX_POINT('',#97813);
#9765=VERTEX_POINT('',#97815);
#9766=VERTEX_POINT('',#97820);
#9767=VERTEX_POINT('',#97822);
#9768=VERTEX_POINT('',#97824);
#9769=VERTEX_POINT('',#97828);
#9770=VERTEX_POINT('',#97830);
#9771=VERTEX_POINT('',#97843);
#9772=VERTEX_POINT('',#97845);
#9773=VERTEX_POINT('',#97849);
#9774=VERTEX_POINT('',#97853);
#9775=VERTEX_POINT('',#97857);
#9776=VERTEX_POINT('',#97859);
#9777=VERTEX_POINT('',#97888);
#9778=VERTEX_POINT('',#97916);
#9779=VERTEX_POINT('',#97918);
#9780=VERTEX_POINT('',#97922);
#9781=VERTEX_POINT('',#97926);
#9782=VERTEX_POINT('',#97928);
#9783=VERTEX_POINT('',#97930);
#9784=VERTEX_POINT('',#97936);
#9785=VERTEX_POINT('',#98082);
#9786=VERTEX_POINT('',#98252);
#9787=VERTEX_POINT('',#98280);
#9788=VERTEX_POINT('',#98291);
#9789=VERTEX_POINT('',#98296);
#9790=VERTEX_POINT('',#98310);
#9791=VERTEX_POINT('',#98312);
#9792=VERTEX_POINT('',#98314);
#9793=VERTEX_POINT('',#98319);
#9794=VERTEX_POINT('',#98324);
#9795=VERTEX_POINT('',#98486);
#9796=VERTEX_POINT('',#98516);
#9797=VERTEX_POINT('',#98547);
#9798=VERTEX_POINT('',#98549);
#9799=VERTEX_POINT('',#98552);
#9800=VERTEX_POINT('',#98554);
#9801=VERTEX_POINT('',#98706);
#9802=VERTEX_POINT('',#98877);
#9803=VERTEX_POINT('',#98904);
#9804=VERTEX_POINT('',#98909);
#9805=VERTEX_POINT('',#98932);
#9806=VERTEX_POINT('',#98937);
#9807=VERTEX_POINT('',#98951);
#9808=VERTEX_POINT('',#98953);
#9809=VERTEX_POINT('',#98955);
#9810=VERTEX_POINT('',#98969);
#9811=VERTEX_POINT('',#99135);
#9812=VERTEX_POINT('',#99161);
#9813=VERTEX_POINT('',#99187);
#9814=VERTEX_POINT('',#99223);
#9815=VERTEX_POINT('',#99247);
#9816=VERTEX_POINT('',#99249);
#9817=VERTEX_POINT('',#99253);
#9818=VERTEX_POINT('',#99254);
#9819=VERTEX_POINT('',#99260);
#9820=VERTEX_POINT('',#99298);
#9821=VERTEX_POINT('',#99300);
#9822=VERTEX_POINT('',#99362);
#9823=VERTEX_POINT('',#99393);
#9824=VERTEX_POINT('',#99395);
#9825=VERTEX_POINT('',#99397);
#9826=VERTEX_POINT('',#99399);
#9827=VERTEX_POINT('',#99401);
#9828=VERTEX_POINT('',#99403);
#9829=VERTEX_POINT('',#99425);
#9830=VERTEX_POINT('',#99429);
#9831=VERTEX_POINT('',#99442);
#9832=VERTEX_POINT('',#99449);
#9833=VERTEX_POINT('',#99451);
#9834=VERTEX_POINT('',#99453);
#9835=VERTEX_POINT('',#99478);
#9836=VERTEX_POINT('',#99546);
#9837=VERTEX_POINT('',#99639);
#9838=VERTEX_POINT('',#99641);
#9839=VERTEX_POINT('',#99644);
#9840=VERTEX_POINT('',#99646);
#9841=VERTEX_POINT('',#99650);
#9842=VERTEX_POINT('',#99652);
#9843=VERTEX_POINT('',#99658);
#9844=VERTEX_POINT('',#99660);
#9845=VERTEX_POINT('',#99664);
#9846=VERTEX_POINT('',#99666);
#9847=VERTEX_POINT('',#99670);
#9848=VERTEX_POINT('',#99675);
#9849=VERTEX_POINT('',#99678);
#9850=VERTEX_POINT('',#99680);
#9851=VERTEX_POINT('',#99684);
#9852=VERTEX_POINT('',#99686);
#9853=VERTEX_POINT('',#99692);
#9854=VERTEX_POINT('',#99694);
#9855=VERTEX_POINT('',#99698);
#9856=VERTEX_POINT('',#99700);
#12625=EDGE_CURVE('',#9759,#9760,#1035,.T.);
#12626=EDGE_CURVE('',#9760,#9761,#3183,.T.);
#12627=EDGE_CURVE('',#9761,#9762,#1036,.T.);
#12628=EDGE_CURVE('',#9762,#9759,#3184,.T.);
#12629=EDGE_CURVE('',#9763,#9764,#1037,.T.);
#12630=EDGE_CURVE('',#9764,#9765,#3185,.T.);
#12631=EDGE_CURVE('',#9765,#9761,#1038,.T.);
#12632=EDGE_CURVE('',#9761,#9763,#3186,.T.);
#12633=EDGE_CURVE('',#9766,#9763,#1039,.T.);
#12634=EDGE_CURVE('',#9763,#9767,#3187,.T.);
#12635=EDGE_CURVE('',#9767,#9768,#1040,.T.);
#12636=EDGE_CURVE('',#9768,#9766,#3188,.T.);
#12637=EDGE_CURVE('',#9760,#9769,#1041,.T.);
#12638=EDGE_CURVE('',#9769,#9770,#3189,.T.);
#12639=EDGE_CURVE('',#9770,#9767,#1042,.T.);
#12640=EDGE_CURVE('',#9767,#9760,#3190,.T.);
#12641=EDGE_CURVE('',#9770,#9768,#1043,.T.);
#12642=EDGE_CURVE('',#9766,#9764,#1044,.T.);
#12643=EDGE_CURVE('',#9765,#9762,#1045,.T.);
#12644=EDGE_CURVE('',#9759,#9769,#1046,.T.);
#12645=EDGE_CURVE('',#9766,#9771,#3191,.T.);
#12646=EDGE_CURVE('',#9771,#9772,#1047,.T.);
#12647=EDGE_CURVE('',#9772,#9764,#3192,.T.);
#12648=EDGE_CURVE('',#9773,#9768,#3193,.T.);
#12649=EDGE_CURVE('',#9771,#9773,#3194,.T.);
#12650=EDGE_CURVE('',#9770,#9774,#3195,.T.);
#12651=EDGE_CURVE('',#9774,#9773,#1048,.T.);
#12652=EDGE_CURVE('',#9775,#9769,#3196,.T.);
#12653=EDGE_CURVE('',#9776,#9775,#8003,.T.);
#12654=EDGE_CURVE('',#9777,#9776,#3197,.T.);
#12655=EDGE_CURVE('',#9774,#9777,#8004,.T.);
#12656=EDGE_CURVE('',#9778,#9778,#1049,.T.);
#12657=EDGE_CURVE('',#9779,#9779,#1050,.T.);
#12658=EDGE_CURVE('',#9759,#9780,#3198,.T.);
#12659=EDGE_CURVE('',#9780,#9775,#1051,.T.);
#12660=EDGE_CURVE('',#9781,#9780,#1052,.T.);
#12661=EDGE_CURVE('',#9780,#9782,#3199,.T.);
#12662=EDGE_CURVE('',#9782,#9783,#1053,.T.);
#12663=EDGE_CURVE('',#9783,#9781,#3200,.T.);
#12664=EDGE_CURVE('',#9781,#9775,#1054,.T.);
#12665=EDGE_CURVE('',#9765,#9784,#3201,.T.);
#12666=EDGE_CURVE('',#9784,#9782,#1055,.T.);
#12667=EDGE_CURVE('',#9782,#9762,#3202,.T.);
#12668=EDGE_CURVE('',#9784,#9783,#1056,.T.);
#12669=EDGE_CURVE('',#9781,#9785,#8005,.T.);
#12670=EDGE_CURVE('',#9776,#9785,#1057,.T.);
#12671=EDGE_CURVE('',#9786,#9783,#8006,.T.);
#12672=EDGE_CURVE('',#9787,#9786,#8007,.T.);
#12673=EDGE_CURVE('',#9788,#9787,#8008,.T.);
#12674=EDGE_CURVE('',#9789,#9788,#8009,.T.);
#12675=EDGE_CURVE('',#9790,#9789,#1058,.T.);
#12676=EDGE_CURVE('',#9790,#9791,#3203,.T.);
#12677=EDGE_CURVE('',#9792,#9791,#8010,.T.);
#12678=EDGE_CURVE('',#9793,#9792,#8011,.T.);
#12679=EDGE_CURVE('',#9794,#9793,#8012,.T.);
#12680=EDGE_CURVE('',#9785,#9794,#8013,.T.);
#12681=EDGE_CURVE('',#9784,#9795,#8014,.T.);
#12682=EDGE_CURVE('',#9786,#9795,#1059,.T.);
#12683=EDGE_CURVE('',#9796,#9772,#8015,.T.);
#12684=EDGE_CURVE('',#9795,#9796,#3204,.T.);
#12685=EDGE_CURVE('',#9797,#9797,#1060,.T.);
#12686=EDGE_CURVE('',#9798,#9798,#1061,.T.);
#12687=EDGE_CURVE('',#9773,#9799,#1062,.T.);
#12688=EDGE_CURVE('',#9799,#9800,#3205,.T.);
#12689=EDGE_CURVE('',#9800,#9771,#1063,.T.);
#12690=EDGE_CURVE('',#9774,#9799,#1064,.T.);
#12691=EDGE_CURVE('',#9800,#9772,#1065,.T.);
#12692=EDGE_CURVE('',#9800,#9801,#8016,.T.);
#12693=EDGE_CURVE('',#9796,#9801,#1066,.T.);
#12694=EDGE_CURVE('',#9802,#9799,#8017,.T.);
#12695=EDGE_CURVE('',#9803,#9802,#8018,.T.);
#12696=EDGE_CURVE('',#9804,#9803,#8019,.T.);
#12697=EDGE_CURVE('',#9805,#9804,#8020,.T.);
#12698=EDGE_CURVE('',#9806,#9805,#8021,.T.);
#12699=EDGE_CURVE('',#9807,#9806,#3206,.T.);
#12700=EDGE_CURVE('',#9808,#9807,#1067,.T.);
#12701=EDGE_CURVE('',#9809,#9808,#8022,.T.);
#12702=EDGE_CURVE('',#9810,#9809,#8023,.T.);
#12703=EDGE_CURVE('',#9801,#9810,#8024,.T.);
#12704=EDGE_CURVE('',#9777,#9802,#1068,.T.);
#12705=EDGE_CURVE('',#9777,#9811,#8025,.T.);
#12706=EDGE_CURVE('',#9811,#9803,#1069,.T.);
#12707=EDGE_CURVE('',#9812,#9804,#1070,.T.);
#12708=EDGE_CURVE('',#9811,#9812,#8026,.T.);
#12709=EDGE_CURVE('',#9812,#9813,#8027,.T.);
#12710=EDGE_CURVE('',#9813,#9805,#1071,.T.);
#12711=EDGE_CURVE('',#9813,#9814,#8028,.T.);
#12712=EDGE_CURVE('',#9814,#9806,#8029,.T.);
#12713=EDGE_CURVE('',#9814,#9815,#3207,.T.);
#12714=EDGE_CURVE('',#9815,#9816,#1072,.T.);
#12715=EDGE_CURVE('',#9816,#9806,#3208,.T.);
#12716=EDGE_CURVE('',#9817,#9818,#1073,.T.);
#12717=EDGE_CURVE('',#9818,#9816,#1074,.T.);
#12718=EDGE_CURVE('',#9815,#9817,#1075,.T.);
#12719=EDGE_CURVE('',#9791,#9818,#3209,.T.);
#12720=EDGE_CURVE('',#9817,#9819,#3210,.T.);
#12721=EDGE_CURVE('',#9819,#9791,#8030,.T.);
#12722=EDGE_CURVE('',#9792,#9820,#1076,.T.);
#12723=EDGE_CURVE('',#9820,#9821,#8031,.T.);
#12724=EDGE_CURVE('',#9821,#9793,#1077,.T.);
#12725=EDGE_CURVE('',#9819,#9820,#8032,.T.);
#12726=EDGE_CURVE('',#9822,#9794,#1078,.T.);
#12727=EDGE_CURVE('',#9821,#9822,#8033,.T.);
#12728=EDGE_CURVE('',#9822,#9776,#8034,.T.);
#12729=EDGE_CURVE('',#9823,#9816,#3211,.T.);
#12730=EDGE_CURVE('',#9823,#9824,#3212,.T.);
#12731=EDGE_CURVE('',#9824,#9825,#1079,.T.);
#12732=EDGE_CURVE('',#9825,#9826,#3213,.T.);
#12733=EDGE_CURVE('',#9826,#9827,#1978,.T.);
#12734=EDGE_CURVE('',#9827,#9828,#8035,.T.);
#12735=EDGE_CURVE('',#9828,#9807,#8036,.T.);
#12736=EDGE_CURVE('',#9829,#9818,#3214,.T.);
#12737=EDGE_CURVE('',#9829,#9823,#1080,.T.);
#12738=EDGE_CURVE('',#9830,#9790,#8037,.F.);
#12739=EDGE_CURVE('',#9831,#9830,#8038,.F.);
#12740=EDGE_CURVE('',#9832,#9831,#1979,.F.);
#12741=EDGE_CURVE('',#9832,#9833,#3215,.T.);
#12742=EDGE_CURVE('',#9833,#9834,#1081,.T.);
#12743=EDGE_CURVE('',#9834,#9829,#3216,.T.);
#12744=EDGE_CURVE('',#9831,#9788,#1082,.T.);
#12745=EDGE_CURVE('',#9787,#9835,#1083,.T.);
#12746=EDGE_CURVE('',#9835,#9832,#8039,.T.);
#12747=EDGE_CURVE('',#9830,#9789,#1084,.T.);
#12748=EDGE_CURVE('',#9795,#9835,#8040,.T.);
#12749=EDGE_CURVE('',#9836,#9796,#8041,.T.);
#12750=EDGE_CURVE('',#9836,#9835,#3217,.T.);
#12751=EDGE_CURVE('',#9826,#9836,#8042,.T.);
#12752=EDGE_CURVE('',#9836,#9810,#1085,.T.);
#12753=EDGE_CURVE('',#9809,#9827,#1086,.T.);
#12754=EDGE_CURVE('',#9808,#9828,#1087,.T.);
#12755=EDGE_CURVE('',#9833,#9825,#3218,.T.);
#12756=EDGE_CURVE('',#9824,#9834,#3219,.T.);
#12757=EDGE_CURVE('',#9837,#9837,#1088,.T.);
#12758=EDGE_CURVE('',#9838,#9838,#1089,.T.);
#12759=EDGE_CURVE('',#9797,#9839,#1090,.T.);
#12760=EDGE_CURVE('',#9839,#9840,#1091,.T.);
#12761=EDGE_CURVE('',#9840,#9839,#1092,.T.);
#12762=EDGE_CURVE('',#9840,#9841,#3220,.T.);
#12763=EDGE_CURVE('',#9842,#9841,#1093,.T.);
#12764=EDGE_CURVE('',#9841,#9842,#1094,.T.);
#12765=EDGE_CURVE('',#9778,#9842,#1095,.T.);
#12766=EDGE_CURVE('',#9837,#9843,#1096,.T.);
#12767=EDGE_CURVE('',#9843,#9844,#1097,.T.);
#12768=EDGE_CURVE('',#9844,#9843,#1098,.T.);
#12769=EDGE_CURVE('',#9844,#9845,#3221,.T.);
#12770=EDGE_CURVE('',#9846,#9845,#1099,.T.);
#12771=EDGE_CURVE('',#9845,#9846,#1100,.T.);
#12772=EDGE_CURVE('',#9847,#9847,#1101,.T.);
#12773=EDGE_CURVE('',#9847,#9846,#1102,.T.);
#12774=EDGE_CURVE('',#9820,#9813,#3222,.T.);
#12775=EDGE_CURVE('',#9848,#9848,#1103,.T.);
#12776=EDGE_CURVE('',#9798,#9849,#1104,.T.);
#12777=EDGE_CURVE('',#9849,#9850,#1105,.T.);
#12778=EDGE_CURVE('',#9850,#9849,#1106,.T.);
#12779=EDGE_CURVE('',#9850,#9851,#3223,.T.);
#12780=EDGE_CURVE('',#9852,#9851,#1107,.T.);
#12781=EDGE_CURVE('',#9851,#9852,#1108,.T.);
#12782=EDGE_CURVE('',#9779,#9852,#1109,.T.);
#12783=EDGE_CURVE('',#9838,#9853,#1110,.T.);
#12784=EDGE_CURVE('',#9853,#9854,#1111,.T.);
#12785=EDGE_CURVE('',#9854,#9853,#1112,.T.);
#12786=EDGE_CURVE('',#9854,#9855,#3224,.T.);
#12787=EDGE_CURVE('',#9856,#9855,#1113,.T.);
#12788=EDGE_CURVE('',#9855,#9856,#1114,.T.);
#12789=EDGE_CURVE('',#9848,#9856,#1115,.T.);
#12790=EDGE_CURVE('',#9812,#9821,#3225,.T.);
#12791=EDGE_CURVE('',#9822,#9811,#3226,.T.);
#18301=ORIENTED_EDGE('',*,*,#12625,.T.);
#18302=ORIENTED_EDGE('',*,*,#12626,.T.);
#18303=ORIENTED_EDGE('',*,*,#12627,.T.);
#18304=ORIENTED_EDGE('',*,*,#12628,.T.);
#18305=ORIENTED_EDGE('',*,*,#12629,.T.);
#18306=ORIENTED_EDGE('',*,*,#12630,.T.);
#18307=ORIENTED_EDGE('',*,*,#12631,.T.);
#18308=ORIENTED_EDGE('',*,*,#12632,.T.);
#18309=ORIENTED_EDGE('',*,*,#12633,.T.);
#18310=ORIENTED_EDGE('',*,*,#12634,.T.);
#18311=ORIENTED_EDGE('',*,*,#12635,.T.);
#18312=ORIENTED_EDGE('',*,*,#12636,.T.);
#18313=ORIENTED_EDGE('',*,*,#12637,.T.);
#18314=ORIENTED_EDGE('',*,*,#12638,.T.);
#18315=ORIENTED_EDGE('',*,*,#12639,.T.);
#18316=ORIENTED_EDGE('',*,*,#12640,.T.);
#18317=ORIENTED_EDGE('',*,*,#12639,.F.);
#18318=ORIENTED_EDGE('',*,*,#12641,.T.);
#18319=ORIENTED_EDGE('',*,*,#12635,.F.);
#18320=ORIENTED_EDGE('',*,*,#12633,.F.);
#18321=ORIENTED_EDGE('',*,*,#12642,.T.);
#18322=ORIENTED_EDGE('',*,*,#12629,.F.);
#18323=ORIENTED_EDGE('',*,*,#12631,.F.);
#18324=ORIENTED_EDGE('',*,*,#12643,.T.);
#18325=ORIENTED_EDGE('',*,*,#12627,.F.);
#18326=ORIENTED_EDGE('',*,*,#12625,.F.);
#18327=ORIENTED_EDGE('',*,*,#12644,.T.);
#18328=ORIENTED_EDGE('',*,*,#12637,.F.);
#18329=ORIENTED_EDGE('',*,*,#12642,.F.);
#18330=ORIENTED_EDGE('',*,*,#12645,.T.);
#18331=ORIENTED_EDGE('',*,*,#12646,.T.);
#18332=ORIENTED_EDGE('',*,*,#12647,.T.);
#18333=ORIENTED_EDGE('',*,*,#12636,.F.);
#18334=ORIENTED_EDGE('',*,*,#12648,.F.);
#18335=ORIENTED_EDGE('',*,*,#12649,.F.);
#18336=ORIENTED_EDGE('',*,*,#12645,.F.);
#18337=ORIENTED_EDGE('',*,*,#12641,.F.);
#18338=ORIENTED_EDGE('',*,*,#12650,.T.);
#18339=ORIENTED_EDGE('',*,*,#12651,.T.);
#18340=ORIENTED_EDGE('',*,*,#12648,.T.);
#18341=ORIENTED_EDGE('',*,*,#12638,.F.);
#18342=ORIENTED_EDGE('',*,*,#12652,.F.);
#18343=ORIENTED_EDGE('',*,*,#12653,.F.);
#18344=ORIENTED_EDGE('',*,*,#12654,.F.);
#18345=ORIENTED_EDGE('',*,*,#12655,.F.);
#18346=ORIENTED_EDGE('',*,*,#12650,.F.);
#18347=ORIENTED_EDGE('',*,*,#12656,.F.);
#18348=ORIENTED_EDGE('',*,*,#12657,.F.);
#18349=ORIENTED_EDGE('',*,*,#12626,.F.);
#18350=ORIENTED_EDGE('',*,*,#12640,.F.);
#18351=ORIENTED_EDGE('',*,*,#12634,.F.);
#18352=ORIENTED_EDGE('',*,*,#12632,.F.);
#18353=ORIENTED_EDGE('',*,*,#12644,.F.);
#18354=ORIENTED_EDGE('',*,*,#12658,.T.);
#18355=ORIENTED_EDGE('',*,*,#12659,.T.);
#18356=ORIENTED_EDGE('',*,*,#12652,.T.);
#18357=ORIENTED_EDGE('',*,*,#12660,.T.);
#18358=ORIENTED_EDGE('',*,*,#12661,.T.);
#18359=ORIENTED_EDGE('',*,*,#12662,.T.);
#18360=ORIENTED_EDGE('',*,*,#12663,.T.);
#18361=ORIENTED_EDGE('',*,*,#12660,.F.);
#18362=ORIENTED_EDGE('',*,*,#12664,.T.);
#18363=ORIENTED_EDGE('',*,*,#12659,.F.);
#18364=ORIENTED_EDGE('',*,*,#12643,.F.);
#18365=ORIENTED_EDGE('',*,*,#12665,.T.);
#18366=ORIENTED_EDGE('',*,*,#12666,.T.);
#18367=ORIENTED_EDGE('',*,*,#12667,.T.);
#18368=ORIENTED_EDGE('',*,*,#12666,.F.);
#18369=ORIENTED_EDGE('',*,*,#12668,.T.);
#18370=ORIENTED_EDGE('',*,*,#12662,.F.);
#18371=ORIENTED_EDGE('',*,*,#12664,.F.);
#18372=ORIENTED_EDGE('',*,*,#12669,.T.);
#18373=ORIENTED_EDGE('',*,*,#12670,.F.);
#18374=ORIENTED_EDGE('',*,*,#12653,.T.);
#18375=ORIENTED_EDGE('',*,*,#12663,.F.);
#18376=ORIENTED_EDGE('',*,*,#12671,.F.);
#18377=ORIENTED_EDGE('',*,*,#12672,.F.);
#18378=ORIENTED_EDGE('',*,*,#12673,.F.);
#18379=ORIENTED_EDGE('',*,*,#12674,.F.);
#18380=ORIENTED_EDGE('',*,*,#12675,.F.);
#18381=ORIENTED_EDGE('',*,*,#12676,.T.);
#18382=ORIENTED_EDGE('',*,*,#12677,.F.);
#18383=ORIENTED_EDGE('',*,*,#12678,.F.);
#18384=ORIENTED_EDGE('',*,*,#12679,.F.);
#18385=ORIENTED_EDGE('',*,*,#12680,.F.);
#18386=ORIENTED_EDGE('',*,*,#12669,.F.);
#18387=ORIENTED_EDGE('',*,*,#12668,.F.);
#18388=ORIENTED_EDGE('',*,*,#12681,.T.);
#18389=ORIENTED_EDGE('',*,*,#12682,.F.);
#18390=ORIENTED_EDGE('',*,*,#12671,.T.);
#18391=ORIENTED_EDGE('',*,*,#12630,.F.);
#18392=ORIENTED_EDGE('',*,*,#12647,.F.);
#18393=ORIENTED_EDGE('',*,*,#12683,.F.);
#18394=ORIENTED_EDGE('',*,*,#12684,.F.);
#18395=ORIENTED_EDGE('',*,*,#12681,.F.);
#18396=ORIENTED_EDGE('',*,*,#12665,.F.);
#18397=ORIENTED_EDGE('',*,*,#12685,.F.);
#18398=ORIENTED_EDGE('',*,*,#12686,.F.);
#18399=ORIENTED_EDGE('',*,*,#12687,.T.);
#18400=ORIENTED_EDGE('',*,*,#12688,.T.);
#18401=ORIENTED_EDGE('',*,*,#12689,.T.);
#18402=ORIENTED_EDGE('',*,*,#12649,.T.);
#18403=ORIENTED_EDGE('',*,*,#12651,.F.);
#18404=ORIENTED_EDGE('',*,*,#12690,.T.);
#18405=ORIENTED_EDGE('',*,*,#12687,.F.);
#18406=ORIENTED_EDGE('',*,*,#12689,.F.);
#18407=ORIENTED_EDGE('',*,*,#12691,.T.);
#18408=ORIENTED_EDGE('',*,*,#12646,.F.);
#18409=ORIENTED_EDGE('',*,*,#12691,.F.);
#18410=ORIENTED_EDGE('',*,*,#12692,.T.);
#18411=ORIENTED_EDGE('',*,*,#12693,.F.);
#18412=ORIENTED_EDGE('',*,*,#12683,.T.);
#18413=ORIENTED_EDGE('',*,*,#12688,.F.);
#18414=ORIENTED_EDGE('',*,*,#12694,.F.);
#18415=ORIENTED_EDGE('',*,*,#12695,.F.);
#18416=ORIENTED_EDGE('',*,*,#12696,.F.);
#18417=ORIENTED_EDGE('',*,*,#12697,.F.);
#18418=ORIENTED_EDGE('',*,*,#12698,.F.);
#18419=ORIENTED_EDGE('',*,*,#12699,.F.);
#18420=ORIENTED_EDGE('',*,*,#12700,.F.);
#18421=ORIENTED_EDGE('',*,*,#12701,.F.);
#18422=ORIENTED_EDGE('',*,*,#12702,.F.);
#18423=ORIENTED_EDGE('',*,*,#12703,.F.);
#18424=ORIENTED_EDGE('',*,*,#12692,.F.);
#18425=ORIENTED_EDGE('',*,*,#12690,.F.);
#18426=ORIENTED_EDGE('',*,*,#12655,.T.);
#18427=ORIENTED_EDGE('',*,*,#12704,.T.);
#18428=ORIENTED_EDGE('',*,*,#12694,.T.);
#18429=ORIENTED_EDGE('',*,*,#12704,.F.);
#18430=ORIENTED_EDGE('',*,*,#12705,.T.);
#18431=ORIENTED_EDGE('',*,*,#12706,.T.);
#18432=ORIENTED_EDGE('',*,*,#12695,.T.);
#18433=ORIENTED_EDGE('',*,*,#12707,.T.);
#18434=ORIENTED_EDGE('',*,*,#12696,.T.);
#18435=ORIENTED_EDGE('',*,*,#12706,.F.);
#18436=ORIENTED_EDGE('',*,*,#12708,.T.);
#18437=ORIENTED_EDGE('',*,*,#12707,.F.);
#18438=ORIENTED_EDGE('',*,*,#12709,.T.);
#18439=ORIENTED_EDGE('',*,*,#12710,.T.);
#18440=ORIENTED_EDGE('',*,*,#12697,.T.);
#18441=ORIENTED_EDGE('',*,*,#12698,.T.);
#18442=ORIENTED_EDGE('',*,*,#12710,.F.);
#18443=ORIENTED_EDGE('',*,*,#12711,.T.);
#18444=ORIENTED_EDGE('',*,*,#12712,.T.);
#18445=ORIENTED_EDGE('',*,*,#12713,.T.);
#18446=ORIENTED_EDGE('',*,*,#12714,.T.);
#18447=ORIENTED_EDGE('',*,*,#12715,.T.);
#18448=ORIENTED_EDGE('',*,*,#12712,.F.);
#18449=ORIENTED_EDGE('',*,*,#12716,.T.);
#18450=ORIENTED_EDGE('',*,*,#12717,.T.);
#18451=ORIENTED_EDGE('',*,*,#12714,.F.);
#18452=ORIENTED_EDGE('',*,*,#12718,.T.);
#18453=ORIENTED_EDGE('',*,*,#12719,.T.);
#18454=ORIENTED_EDGE('',*,*,#12716,.F.);
#18455=ORIENTED_EDGE('',*,*,#12720,.T.);
#18456=ORIENTED_EDGE('',*,*,#12721,.T.);
#18457=ORIENTED_EDGE('',*,*,#12722,.T.);
#18458=ORIENTED_EDGE('',*,*,#12723,.T.);
#18459=ORIENTED_EDGE('',*,*,#12724,.T.);
#18460=ORIENTED_EDGE('',*,*,#12678,.T.);
#18461=ORIENTED_EDGE('',*,*,#12725,.T.);
#18462=ORIENTED_EDGE('',*,*,#12722,.F.);
#18463=ORIENTED_EDGE('',*,*,#12677,.T.);
#18464=ORIENTED_EDGE('',*,*,#12721,.F.);
#18465=ORIENTED_EDGE('',*,*,#12726,.T.);
#18466=ORIENTED_EDGE('',*,*,#12679,.T.);
#18467=ORIENTED_EDGE('',*,*,#12724,.F.);
#18468=ORIENTED_EDGE('',*,*,#12727,.T.);
#18469=ORIENTED_EDGE('',*,*,#12726,.F.);
#18470=ORIENTED_EDGE('',*,*,#12728,.T.);
#18471=ORIENTED_EDGE('',*,*,#12670,.T.);
#18472=ORIENTED_EDGE('',*,*,#12680,.T.);
#18473=ORIENTED_EDGE('',*,*,#12715,.F.);
#18474=ORIENTED_EDGE('',*,*,#12729,.F.);
#18475=ORIENTED_EDGE('',*,*,#12730,.T.);
#18476=ORIENTED_EDGE('',*,*,#12731,.T.);
#18477=ORIENTED_EDGE('',*,*,#12732,.T.);
#18478=ORIENTED_EDGE('',*,*,#12733,.T.);
#18479=ORIENTED_EDGE('',*,*,#12734,.T.);
#18480=ORIENTED_EDGE('',*,*,#12735,.T.);
#18481=ORIENTED_EDGE('',*,*,#12699,.T.);
#18482=ORIENTED_EDGE('',*,*,#12717,.F.);
#18483=ORIENTED_EDGE('',*,*,#12736,.F.);
#18484=ORIENTED_EDGE('',*,*,#12737,.T.);
#18485=ORIENTED_EDGE('',*,*,#12729,.T.);
#18486=ORIENTED_EDGE('',*,*,#12719,.F.);
#18487=ORIENTED_EDGE('',*,*,#12676,.F.);
#18488=ORIENTED_EDGE('',*,*,#12738,.F.);
#18489=ORIENTED_EDGE('',*,*,#12739,.F.);
#18490=ORIENTED_EDGE('',*,*,#12740,.F.);
#18491=ORIENTED_EDGE('',*,*,#12741,.T.);
#18492=ORIENTED_EDGE('',*,*,#12742,.T.);
#18493=ORIENTED_EDGE('',*,*,#12743,.T.);
#18494=ORIENTED_EDGE('',*,*,#12736,.T.);
#18495=ORIENTED_EDGE('',*,*,#12628,.F.);
#18496=ORIENTED_EDGE('',*,*,#12667,.F.);
#18497=ORIENTED_EDGE('',*,*,#12661,.F.);
#18498=ORIENTED_EDGE('',*,*,#12658,.F.);
#18499=ORIENTED_EDGE('',*,*,#12740,.T.);
#18500=ORIENTED_EDGE('',*,*,#12744,.T.);
#18501=ORIENTED_EDGE('',*,*,#12673,.T.);
#18502=ORIENTED_EDGE('',*,*,#12745,.T.);
#18503=ORIENTED_EDGE('',*,*,#12746,.T.);
#18504=ORIENTED_EDGE('',*,*,#12739,.T.);
#18505=ORIENTED_EDGE('',*,*,#12747,.T.);
#18506=ORIENTED_EDGE('',*,*,#12674,.T.);
#18507=ORIENTED_EDGE('',*,*,#12744,.F.);
#18508=ORIENTED_EDGE('',*,*,#12738,.T.);
#18509=ORIENTED_EDGE('',*,*,#12675,.T.);
#18510=ORIENTED_EDGE('',*,*,#12747,.F.);
#18511=ORIENTED_EDGE('',*,*,#12682,.T.);
#18512=ORIENTED_EDGE('',*,*,#12748,.T.);
#18513=ORIENTED_EDGE('',*,*,#12745,.F.);
#18514=ORIENTED_EDGE('',*,*,#12672,.T.);
#18515=ORIENTED_EDGE('',*,*,#12748,.F.);
#18516=ORIENTED_EDGE('',*,*,#12684,.T.);
#18517=ORIENTED_EDGE('',*,*,#12749,.F.);
#18518=ORIENTED_EDGE('',*,*,#12750,.T.);
#18519=ORIENTED_EDGE('',*,*,#12733,.F.);
#18520=ORIENTED_EDGE('',*,*,#12751,.T.);
#18521=ORIENTED_EDGE('',*,*,#12752,.T.);
#18522=ORIENTED_EDGE('',*,*,#12702,.T.);
#18523=ORIENTED_EDGE('',*,*,#12753,.T.);
#18524=ORIENTED_EDGE('',*,*,#12752,.F.);
#18525=ORIENTED_EDGE('',*,*,#12749,.T.);
#18526=ORIENTED_EDGE('',*,*,#12693,.T.);
#18527=ORIENTED_EDGE('',*,*,#12703,.T.);
#18528=ORIENTED_EDGE('',*,*,#12734,.F.);
#18529=ORIENTED_EDGE('',*,*,#12753,.F.);
#18530=ORIENTED_EDGE('',*,*,#12701,.T.);
#18531=ORIENTED_EDGE('',*,*,#12754,.T.);
#18532=ORIENTED_EDGE('',*,*,#12735,.F.);
#18533=ORIENTED_EDGE('',*,*,#12754,.F.);
#18534=ORIENTED_EDGE('',*,*,#12700,.T.);
#18535=ORIENTED_EDGE('',*,*,#12742,.F.);
#18536=ORIENTED_EDGE('',*,*,#12755,.T.);
#18537=ORIENTED_EDGE('',*,*,#12731,.F.);
#18538=ORIENTED_EDGE('',*,*,#12756,.T.);
#18539=ORIENTED_EDGE('',*,*,#12743,.F.);
#18540=ORIENTED_EDGE('',*,*,#12756,.F.);
#18541=ORIENTED_EDGE('',*,*,#12730,.F.);
#18542=ORIENTED_EDGE('',*,*,#12737,.F.);
#18543=ORIENTED_EDGE('',*,*,#12757,.F.);
#18544=ORIENTED_EDGE('',*,*,#12758,.F.);
#18545=ORIENTED_EDGE('',*,*,#12685,.T.);
#18546=ORIENTED_EDGE('',*,*,#12759,.T.);
#18547=ORIENTED_EDGE('',*,*,#12760,.T.);
#18548=ORIENTED_EDGE('',*,*,#12761,.T.);
#18549=ORIENTED_EDGE('',*,*,#12759,.F.);
#18550=ORIENTED_EDGE('',*,*,#12761,.F.);
#18551=ORIENTED_EDGE('',*,*,#12762,.T.);
#18552=ORIENTED_EDGE('',*,*,#12763,.F.);
#18553=ORIENTED_EDGE('',*,*,#12764,.F.);
#18554=ORIENTED_EDGE('',*,*,#12762,.F.);
#18555=ORIENTED_EDGE('',*,*,#12760,.F.);
#18556=ORIENTED_EDGE('',*,*,#12656,.T.);
#18557=ORIENTED_EDGE('',*,*,#12765,.T.);
#18558=ORIENTED_EDGE('',*,*,#12763,.T.);
#18559=ORIENTED_EDGE('',*,*,#12764,.T.);
#18560=ORIENTED_EDGE('',*,*,#12765,.F.);
#18561=ORIENTED_EDGE('',*,*,#12757,.T.);
#18562=ORIENTED_EDGE('',*,*,#12766,.T.);
#18563=ORIENTED_EDGE('',*,*,#12767,.T.);
#18564=ORIENTED_EDGE('',*,*,#12768,.T.);
#18565=ORIENTED_EDGE('',*,*,#12766,.F.);
#18566=ORIENTED_EDGE('',*,*,#12768,.F.);
#18567=ORIENTED_EDGE('',*,*,#12769,.T.);
#18568=ORIENTED_EDGE('',*,*,#12770,.F.);
#18569=ORIENTED_EDGE('',*,*,#12771,.F.);
#18570=ORIENTED_EDGE('',*,*,#12769,.F.);
#18571=ORIENTED_EDGE('',*,*,#12767,.F.);
#18572=ORIENTED_EDGE('',*,*,#12772,.T.);
#18573=ORIENTED_EDGE('',*,*,#12773,.T.);
#18574=ORIENTED_EDGE('',*,*,#12770,.T.);
#18575=ORIENTED_EDGE('',*,*,#12771,.T.);
#18576=ORIENTED_EDGE('',*,*,#12773,.F.);
#18577=ORIENTED_EDGE('',*,*,#12711,.F.);
#18578=ORIENTED_EDGE('',*,*,#12774,.F.);
#18579=ORIENTED_EDGE('',*,*,#12725,.F.);
#18580=ORIENTED_EDGE('',*,*,#12720,.F.);
#18581=ORIENTED_EDGE('',*,*,#12718,.F.);
#18582=ORIENTED_EDGE('',*,*,#12713,.F.);
#18583=ORIENTED_EDGE('',*,*,#12775,.F.);
#18584=ORIENTED_EDGE('',*,*,#12772,.F.);
#18585=ORIENTED_EDGE('',*,*,#12686,.T.);
#18586=ORIENTED_EDGE('',*,*,#12776,.T.);
#18587=ORIENTED_EDGE('',*,*,#12777,.T.);
#18588=ORIENTED_EDGE('',*,*,#12778,.T.);
#18589=ORIENTED_EDGE('',*,*,#12776,.F.);
#18590=ORIENTED_EDGE('',*,*,#12778,.F.);
#18591=ORIENTED_EDGE('',*,*,#12779,.T.);
#18592=ORIENTED_EDGE('',*,*,#12780,.F.);
#18593=ORIENTED_EDGE('',*,*,#12781,.F.);
#18594=ORIENTED_EDGE('',*,*,#12779,.F.);
#18595=ORIENTED_EDGE('',*,*,#12777,.F.);
#18596=ORIENTED_EDGE('',*,*,#12657,.T.);
#18597=ORIENTED_EDGE('',*,*,#12782,.T.);
#18598=ORIENTED_EDGE('',*,*,#12780,.T.);
#18599=ORIENTED_EDGE('',*,*,#12781,.T.);
#18600=ORIENTED_EDGE('',*,*,#12782,.F.);
#18601=ORIENTED_EDGE('',*,*,#12758,.T.);
#18602=ORIENTED_EDGE('',*,*,#12783,.T.);
#18603=ORIENTED_EDGE('',*,*,#12784,.T.);
#18604=ORIENTED_EDGE('',*,*,#12785,.T.);
#18605=ORIENTED_EDGE('',*,*,#12783,.F.);
#18606=ORIENTED_EDGE('',*,*,#12785,.F.);
#18607=ORIENTED_EDGE('',*,*,#12786,.T.);
#18608=ORIENTED_EDGE('',*,*,#12787,.F.);
#18609=ORIENTED_EDGE('',*,*,#12788,.F.);
#18610=ORIENTED_EDGE('',*,*,#12786,.F.);
#18611=ORIENTED_EDGE('',*,*,#12784,.F.);
#18612=ORIENTED_EDGE('',*,*,#12775,.T.);
#18613=ORIENTED_EDGE('',*,*,#12789,.T.);
#18614=ORIENTED_EDGE('',*,*,#12787,.T.);
#18615=ORIENTED_EDGE('',*,*,#12788,.T.);
#18616=ORIENTED_EDGE('',*,*,#12789,.F.);
#18617=ORIENTED_EDGE('',*,*,#12746,.F.);
#18618=ORIENTED_EDGE('',*,*,#12750,.F.);
#18619=ORIENTED_EDGE('',*,*,#12751,.F.);
#18620=ORIENTED_EDGE('',*,*,#12732,.F.);
#18621=ORIENTED_EDGE('',*,*,#12755,.F.);
#18622=ORIENTED_EDGE('',*,*,#12741,.F.);
#18623=ORIENTED_EDGE('',*,*,#12709,.F.);
#18624=ORIENTED_EDGE('',*,*,#12790,.T.);
#18625=ORIENTED_EDGE('',*,*,#12723,.F.);
#18626=ORIENTED_EDGE('',*,*,#12774,.T.);
#18627=ORIENTED_EDGE('',*,*,#12705,.F.);
#18628=ORIENTED_EDGE('',*,*,#12654,.T.);
#18629=ORIENTED_EDGE('',*,*,#12728,.F.);
#18630=ORIENTED_EDGE('',*,*,#12791,.T.);
#18631=ORIENTED_EDGE('',*,*,#12708,.F.);
#18632=ORIENTED_EDGE('',*,*,#12791,.F.);
#18633=ORIENTED_EDGE('',*,*,#12727,.F.);
#18634=ORIENTED_EDGE('',*,*,#12790,.F.);
#18938=B_SPLINE_SURFACE_WITH_KNOTS('',3,3,((#97942,#97943,#97944,#97945,
#97946,#97947,#97948,#97949,#97950,#97951,#97952,#97953,#97954,#97955,#97956,
#97957,#97958,#97959,#97960,#97961,#97962,#97963,#97964,#97965,#97966,#97967,
#97968,#97969),(#97970,#97971,#97972,#97973,#97974,#97975,#97976,#97977,
#97978,#97979,#97980,#97981,#97982,#97983,#97984,#97985,#97986,#97987,#97988,
#97989,#97990,#97991,#97992,#97993,#97994,#97995,#97996,#97997),(#97998,
#97999,#98000,#98001,#98002,#98003,#98004,#98005,#98006,#98007,#98008,#98009,
#98010,#98011,#98012,#98013,#98014,#98015,#98016,#98017,#98018,#98019,#98020,
#98021,#98022,#98023,#98024,#98025),(#98026,#98027,#98028,#98029,#98030,
#98031,#98032,#98033,#98034,#98035,#98036,#98037,#98038,#98039,#98040,#98041,
#98042,#98043,#98044,#98045,#98046,#98047,#98048,#98049,#98050,#98051,#98052,
#98053),(#98054,#98055,#98056,#98057,#98058,#98059,#98060,#98061,#98062,
#98063,#98064,#98065,#98066,#98067,#98068,#98069,#98070,#98071,#98072,#98073,
#98074,#98075,#98076,#98077,#98078,#98079,#98080,#98081)),.UNSPECIFIED.,
 .F.,.F.,.F.,(4,1,4),(4,1,1,1,1,1,1,1,1,1,1,1,1,1,1,1,1,1,1,1,1,1,1,1,1,
4),(0.,0.5,1.),(3.41679525229117E-14,0.241483590676928,0.482967181353822,
0.96593436270761,1.2074179533845,1.4489015440614,1.69038513473829,1.81112693007674,
1.87149782774596,1.90168327658057,1.93186872541519,2.05261052075363,2.11298141842286,
2.17335231609208,2.2337232137613,2.29409411143053,2.35446500909975,2.41483590676897,
2.53557770210742,2.65631949744587,2.77706129278432,2.89780308812276,3.01854488346121,
3.13928667879966,3.2600284741381,3.38077026947655),.UNSPECIFIED.);
#18939=B_SPLINE_SURFACE_WITH_KNOTS('',5,1,((#98112,#98113),(#98114,#98115),
(#98116,#98117),(#98118,#98119),(#98120,#98121),(#98122,#98123),(#98124,
#98125),(#98126,#98127),(#98128,#98129),(#98130,#98131),(#98132,#98133),
(#98134,#98135),(#98136,#98137),(#98138,#98139),(#98140,#98141),(#98142,
#98143),(#98144,#98145),(#98146,#98147),(#98148,#98149),(#98150,#98151),
(#98152,#98153),(#98154,#98155),(#98156,#98157),(#98158,#98159),(#98160,
#98161),(#98162,#98163),(#98164,#98165),(#98166,#98167),(#98168,#98169),
(#98170,#98171),(#98172,#98173),(#98174,#98175),(#98176,#98177),(#98178,
#98179),(#98180,#98181),(#98182,#98183),(#98184,#98185),(#98186,#98187),
(#98188,#98189),(#98190,#98191),(#98192,#98193),(#98194,#98195),(#98196,
#98197),(#98198,#98199),(#98200,#98201),(#98202,#98203),(#98204,#98205),
(#98206,#98207),(#98208,#98209),(#98210,#98211),(#98212,#98213),(#98214,
#98215),(#98216,#98217),(#98218,#98219),(#98220,#98221),(#98222,#98223),
(#98224,#98225),(#98226,#98227),(#98228,#98229),(#98230,#98231),(#98232,
#98233),(#98234,#98235),(#98236,#98237),(#98238,#98239),(#98240,#98241),
(#98242,#98243),(#98244,#98245),(#98246,#98247),(#98248,#98249),(#98250,
#98251)),.UNSPECIFIED.,.F.,.F.,.F.,(6,1,1,1,1,1,1,1,1,1,1,1,1,1,1,1,1,1,
1,1,1,1,1,1,1,1,1,1,1,1,1,1,1,1,1,1,1,1,1,1,1,1,1,1,1,1,1,1,1,1,1,1,1,1,
1,1,1,1,1,1,1,1,1,1,1,6),(2,2),(0.,0.0153846153846154,0.0307692307692308,
0.0461538461538462,0.0615384615384615,0.0769230769230769,0.0923076923076923,
0.107692307692308,0.123076923076923,0.138461538461538,0.153846153846154,
0.169230769230769,0.184615384615385,0.2,0.215384615384615,0.230769230769231,
0.246153846153846,0.261538461538462,0.276923076923077,0.292307692307692,
0.307692307692308,0.323076923076923,0.338461538461538,0.353846153846154,
0.369230769230769,0.384615384615385,0.4,0.415384615384615,0.430769230769231,
0.446153846153846,0.461538461538462,0.476923076923077,0.492307692307692,
0.507692307692308,0.523076923076923,0.538461538461538,0.553846153846154,
0.569230769230769,0.584615384615384,0.6,0.615384615384615,0.63076923076923,
0.646153846153846,0.661538461538461,0.676923076923076,0.692307692307692,
0.707692307692307,0.723076923076922,0.738461538461538,0.753846153846153,
0.769230769230768,0.784615384615384,0.799999999999999,0.815384615384614,
0.83076923076923,0.846153846153845,0.86153846153846,0.876923076923076,0.892307692307691,
0.907692307692306,0.923076923076922,0.938461538461537,0.953846153846152,
0.969230769230768,0.984615384615383,1.),(0.,1.4688),.UNSPECIFIED.);
#18940=B_SPLINE_SURFACE_WITH_KNOTS('',3,3,((#98351,#98352,#98353,#98354,
#98355,#98356,#98357,#98358,#98359,#98360,#98361,#98362,#98363,#98364,#98365,
#98366,#98367,#98368,#98369,#98370,#98371,#98372,#98373,#98374,#98375,#98376,
#98377),(#98378,#98379,#98380,#98381,#98382,#98383,#98384,#98385,#98386,
#98387,#98388,#98389,#98390,#98391,#98392,#98393,#98394,#98395,#98396,#98397,
#98398,#98399,#98400,#98401,#98402,#98403,#98404),(#98405,#98406,#98407,
#98408,#98409,#98410,#98411,#98412,#98413,#98414,#98415,#98416,#98417,#98418,
#98419,#98420,#98421,#98422,#98423,#98424,#98425,#98426,#98427,#98428,#98429,
#98430,#98431),(#98432,#98433,#98434,#98435,#98436,#98437,#98438,#98439,
#98440,#98441,#98442,#98443,#98444,#98445,#98446,#98447,#98448,#98449,#98450,
#98451,#98452,#98453,#98454,#98455,#98456,#98457,#98458),(#98459,#98460,
#98461,#98462,#98463,#98464,#98465,#98466,#98467,#98468,#98469,#98470,#98471,
#98472,#98473,#98474,#98475,#98476,#98477,#98478,#98479,#98480,#98481,#98482,
#98483,#98484,#98485)),.UNSPECIFIED.,.F.,.F.,.F.,(4,1,4),(4,1,1,1,1,1,1,
1,1,1,1,1,1,1,1,1,1,1,1,1,1,1,1,1,4),(0.,0.5,1.),(0.00128107289438891,0.0623100798183742,
0.12333908674236,0.24539710059033,0.367455114438301,0.489513128286272,0.611571142134242,
0.733629155982213,0.855687169830184,0.977745183678154,1.03877419060214,
1.09980319752612,1.16083220445011,1.1913467079121,1.2218612113741,1.34391922522207,
1.46597723907004,1.71009326676598,1.83215128061395,1.95420929446192,2.19832532215786,
2.4424413498538,2.93067340524569,3.17478943294163,3.41890546063757),
 .UNSPECIFIED.);
#18941=B_SPLINE_SURFACE_WITH_KNOTS('',3,3,((#98561,#98562,#98563,#98564,
#98565,#98566,#98567,#98568,#98569,#98570,#98571,#98572,#98573,#98574,#98575,
#98576,#98577,#98578,#98579,#98580,#98581,#98582,#98583,#98584,#98585,#98586,
#98587,#98588,#98589),(#98590,#98591,#98592,#98593,#98594,#98595,#98596,
#98597,#98598,#98599,#98600,#98601,#98602,#98603,#98604,#98605,#98606,#98607,
#98608,#98609,#98610,#98611,#98612,#98613,#98614,#98615,#98616,#98617,#98618),
(#98619,#98620,#98621,#98622,#98623,#98624,#98625,#98626,#98627,#98628,
#98629,#98630,#98631,#98632,#98633,#98634,#98635,#98636,#98637,#98638,#98639,
#98640,#98641,#98642,#98643,#98644,#98645,#98646,#98647),(#98648,#98649,
#98650,#98651,#98652,#98653,#98654,#98655,#98656,#98657,#98658,#98659,#98660,
#98661,#98662,#98663,#98664,#98665,#98666,#98667,#98668,#98669,#98670,#98671,
#98672,#98673,#98674,#98675,#98676),(#98677,#98678,#98679,#98680,#98681,
#98682,#98683,#98684,#98685,#98686,#98687,#98688,#98689,#98690,#98691,#98692,
#98693,#98694,#98695,#98696,#98697,#98698,#98699,#98700,#98701,#98702,#98703,
#98704,#98705)),.UNSPECIFIED.,.F.,.F.,.F.,(4,1,4),(4,1,1,1,1,1,1,1,1,1,
1,1,1,1,1,1,1,1,1,1,1,1,1,1,1,1,4),(0.,0.5,1.),(0.,0.244116027696041,0.488232055392083,
0.976464110784166,1.22058013848021,1.46469616617625,1.70881219387229,1.83087020772031,
1.89189921464432,1.95292822156833,2.07498623541635,2.13601524234036,2.19704424926437,
2.25807325618838,2.28858775965039,2.31910226311239,2.3801312700364,2.44116027696041,
2.56321829080843,2.68527630465646,2.80733431850448,2.9293923323525,3.05145034620052,
3.17350836004854,3.29556637389656,3.35659538082057,3.41762438774458),
 .UNSPECIFIED.);
#18942=B_SPLINE_SURFACE_WITH_KNOTS('',5,1,((#98737,#98738),(#98739,#98740),
(#98741,#98742),(#98743,#98744),(#98745,#98746),(#98747,#98748),(#98749,
#98750),(#98751,#98752),(#98753,#98754),(#98755,#98756),(#98757,#98758),
(#98759,#98760),(#98761,#98762),(#98763,#98764),(#98765,#98766),(#98767,
#98768),(#98769,#98770),(#98771,#98772),(#98773,#98774),(#98775,#98776),
(#98777,#98778),(#98779,#98780),(#98781,#98782),(#98783,#98784),(#98785,
#98786),(#98787,#98788),(#98789,#98790),(#98791,#98792),(#98793,#98794),
(#98795,#98796),(#98797,#98798),(#98799,#98800),(#98801,#98802),(#98803,
#98804),(#98805,#98806),(#98807,#98808),(#98809,#98810),(#98811,#98812),
(#98813,#98814),(#98815,#98816),(#98817,#98818),(#98819,#98820),(#98821,
#98822),(#98823,#98824),(#98825,#98826),(#98827,#98828),(#98829,#98830),
(#98831,#98832),(#98833,#98834),(#98835,#98836),(#98837,#98838),(#98839,
#98840),(#98841,#98842),(#98843,#98844),(#98845,#98846),(#98847,#98848),
(#98849,#98850),(#98851,#98852),(#98853,#98854),(#98855,#98856),(#98857,
#98858),(#98859,#98860),(#98861,#98862),(#98863,#98864),(#98865,#98866),
(#98867,#98868),(#98869,#98870),(#98871,#98872),(#98873,#98874),(#98875,
#98876)),.UNSPECIFIED.,.F.,.F.,.F.,(6,1,1,1,1,1,1,1,1,1,1,1,1,1,1,1,1,1,
1,1,1,1,1,1,1,1,1,1,1,1,1,1,1,1,1,1,1,1,1,1,1,1,1,1,1,1,1,1,1,1,1,1,1,1,
1,1,1,1,1,1,1,1,1,1,1,6),(2,2),(0.,0.0153846153846154,0.0307692307692308,
0.0461538461538462,0.0615384615384615,0.0769230769230769,0.0923076923076923,
0.107692307692308,0.123076923076923,0.138461538461538,0.153846153846154,
0.169230769230769,0.184615384615385,0.2,0.215384615384615,0.230769230769231,
0.246153846153846,0.261538461538462,0.276923076923077,0.292307692307692,
0.307692307692308,0.323076923076923,0.338461538461538,0.353846153846154,
0.369230769230769,0.384615384615385,0.4,0.415384615384615,0.430769230769231,
0.446153846153846,0.461538461538462,0.476923076923077,0.492307692307692,
0.507692307692308,0.523076923076923,0.538461538461538,0.553846153846154,
0.569230769230769,0.584615384615384,0.6,0.615384615384615,0.63076923076923,
0.646153846153846,0.661538461538461,0.676923076923076,0.692307692307692,
0.707692307692307,0.723076923076922,0.738461538461538,0.753846153846153,
0.769230769230768,0.784615384615384,0.799999999999999,0.815384615384614,
0.83076923076923,0.846153846153845,0.86153846153846,0.876923076923076,0.892307692307691,
0.907692307692306,0.923076923076922,0.938461538461537,0.953846153846152,
0.969230769230768,0.984615384615383,1.),(0.,1.4688),.UNSPECIFIED.);
#18943=B_SPLINE_SURFACE_WITH_KNOTS('',3,3,((#98984,#98985,#98986,#98987,
#98988,#98989,#98990,#98991,#98992,#98993,#98994,#98995,#98996,#98997,#98998,
#98999,#99000,#99001,#99002,#99003,#99004,#99005,#99006,#99007,#99008,#99009),
(#99010,#99011,#99012,#99013,#99014,#99015,#99016,#99017,#99018,#99019,
#99020,#99021,#99022,#99023,#99024,#99025,#99026,#99027,#99028,#99029,#99030,
#99031,#99032,#99033,#99034,#99035),(#99036,#99037,#99038,#99039,#99040,
#99041,#99042,#99043,#99044,#99045,#99046,#99047,#99048,#99049,#99050,#99051,
#99052,#99053,#99054,#99055,#99056,#99057,#99058,#99059,#99060,#99061),
(#99062,#99063,#99064,#99065,#99066,#99067,#99068,#99069,#99070,#99071,
#99072,#99073,#99074,#99075,#99076,#99077,#99078,#99079,#99080,#99081,#99082,
#99083,#99084,#99085,#99086,#99087),(#99088,#99089,#99090,#99091,#99092,
#99093,#99094,#99095,#99096,#99097,#99098,#99099,#99100,#99101,#99102,#99103,
#99104,#99105,#99106,#99107,#99108,#99109,#99110,#99111,#99112,#99113)),
 .UNSPECIFIED.,.F.,.F.,.F.,(4,1,4),(4,1,1,1,1,1,1,1,1,1,1,1,1,1,1,1,1,1,
1,1,1,1,1,4),(0.,0.5,1.),(0.00128110943246098,0.1220229047709,0.242764700109339,
0.363506495447778,0.484248290786216,0.604990086124655,0.725731881463094,
0.846473676801533,0.906844574470752,0.967215472139972,1.02758636980919,
1.08795726747841,1.14832816514763,1.20869906281685,1.26906996048607,1.32944085815529,
1.45018265349373,1.6916662441706,1.93314983484748,2.17463342552436,2.41611701620124,
2.89908419755499,3.14056778823187,3.38205137890875),.UNSPECIFIED.);
#18944=B_SPLINE_SURFACE_WITH_KNOTS('',3,3,((#99115,#99116,#99117,#99118),
(#99119,#99120,#99121,#99122),(#99123,#99124,#99125,#99126),(#99127,#99128,
#99129,#99130),(#99131,#99132,#99133,#99134)),.UNSPECIFIED.,.F.,.F.,.F.,
(4,1,4),(4,4),(0.,0.5,1.),(0.,0.0900415523927057),.UNSPECIFIED.);
#18945=B_SPLINE_SURFACE_WITH_KNOTS('',3,3,((#99141,#99142,#99143,#99144),
(#99145,#99146,#99147,#99148),(#99149,#99150,#99151,#99152),(#99153,#99154,
#99155,#99156),(#99157,#99158,#99159,#99160)),.UNSPECIFIED.,.F.,.F.,.F.,
(4,1,4),(4,4),(0.,0.5,1.00033317135741),(-0.000333171357409007,0.325047276078282),
 .UNSPECIFIED.);
#18946=B_SPLINE_SURFACE_WITH_KNOTS('',3,3,((#99167,#99168,#99169,#99170),
(#99171,#99172,#99173,#99174),(#99175,#99176,#99177,#99178),(#99179,#99180,
#99181,#99182),(#99183,#99184,#99185,#99186)),.UNSPECIFIED.,.F.,.F.,.F.,
(4,1,4),(4,4),(0.,0.5,1.),(0.,0.0523713743724485),.UNSPECIFIED.);
#18947=B_SPLINE_SURFACE_WITH_KNOTS('',3,3,((#99193,#99194,#99195,#99196,
#99197,#99198),(#99199,#99200,#99201,#99202,#99203,#99204),(#99205,#99206,
#99207,#99208,#99209,#99210),(#99211,#99212,#99213,#99214,#99215,#99216),
(#99217,#99218,#99219,#99220,#99221,#99222)),.UNSPECIFIED.,.F.,.F.,.F.,
(4,1,4),(4,2,4),(0.,0.5,1.),(1.22307313571325E-14,0.0771338280521436,0.0784358874721452),
 .UNSPECIFIED.);
#18948=B_SPLINE_SURFACE_WITH_KNOTS('',3,3,((#99278,#99279,#99280,#99281),
(#99282,#99283,#99284,#99285),(#99286,#99287,#99288,#99289),(#99290,#99291,
#99292,#99293),(#99294,#99295,#99296,#99297)),.UNSPECIFIED.,.F.,.F.,.F.,
(4,1,4),(4,4),(0.,0.5,1.),(0.,0.0523726503223924),.UNSPECIFIED.);
#18949=B_SPLINE_SURFACE_WITH_KNOTS('',3,3,((#99306,#99307,#99308,#99309,
#99310,#99311),(#99312,#99313,#99314,#99315,#99316,#99317),(#99318,#99319,
#99320,#99321,#99322,#99323),(#99324,#99325,#99326,#99327,#99328,#99329),
(#99330,#99331,#99332,#99333,#99334,#99335)),.UNSPECIFIED.,.F.,.F.,.F.,
(4,1,4),(4,2,4),(0.,0.5,1.),(-0.00130205941990691,0.,0.0771338280522776),
 .UNSPECIFIED.);
#18950=B_SPLINE_SURFACE_WITH_KNOTS('',3,3,((#99342,#99343,#99344,#99345),
(#99346,#99347,#99348,#99349),(#99350,#99351,#99352,#99353),(#99354,#99355,
#99356,#99357),(#99358,#99359,#99360,#99361)),.UNSPECIFIED.,.F.,.F.,.F.,
(4,1,4),(4,4),(0.,0.5,1.00033317136049),(-0.000333171360490094,0.325047276081303),
 .UNSPECIFIED.);
#18951=B_SPLINE_SURFACE_WITH_KNOTS('',3,3,((#99368,#99369,#99370,#99371),
(#99372,#99373,#99374,#99375),(#99376,#99377,#99378,#99379),(#99380,#99381,
#99382,#99383),(#99384,#99385,#99386,#99387)),.UNSPECIFIED.,.F.,.F.,.F.,
(4,1,4),(4,4),(0.,0.5,1.),(0.,0.0900393973869889),.UNSPECIFIED.);
#18952=B_SPLINE_SURFACE_WITH_KNOTS('',3,3,((#99457,#99458,#99459,#99460),
(#99461,#99462,#99463,#99464),(#99465,#99466,#99467,#99468),(#99469,#99470,
#99471,#99472),(#99473,#99474,#99475,#99476)),.UNSPECIFIED.,.F.,.F.,.F.,
(4,1,4),(4,4),(0.,0.5,1.),(0.,0.324683822128034),.UNSPECIFIED.);
#18953=B_SPLINE_SURFACE_WITH_KNOTS('',3,3,((#99484,#99485,#99486,#99487),
(#99488,#99489,#99490,#99491),(#99492,#99493,#99494,#99495),(#99496,#99497,
#99498,#99499),(#99500,#99501,#99502,#99503)),.UNSPECIFIED.,.F.,.F.,.F.,
(4,1,4),(4,4),(-4.89933240562015E-5,0.309230284442149,0.721537330365014),
(-4.89933240562015E-5,0.0862352312336272),.UNSPECIFIED.);
#18954=B_SPLINE_SURFACE_WITH_KNOTS('',3,3,((#99505,#99506,#99507,#99508),
(#99509,#99510,#99511,#99512),(#99513,#99514,#99515,#99516),(#99517,#99518,
#99519,#99520)),.UNSPECIFIED.,.F.,.F.,.F.,(4,4),(4,4),(0.640913278958594,
1.),(3.45512125000871E-14,0.0441554944102273),.UNSPECIFIED.);
#18955=B_SPLINE_SURFACE_WITH_KNOTS('',3,3,((#99521,#99522,#99523,#99524),
(#99525,#99526,#99527,#99528),(#99529,#99530,#99531,#99532),(#99533,#99534,
#99535,#99536),(#99537,#99538,#99539,#99540)),.UNSPECIFIED.,.F.,.F.,.F.,
(4,1,4),(4,4),(-4.01713313415748E-5,0.5,1.),(-4.01713313414375E-5,0.0546115211509691),
 .UNSPECIFIED.);
#18956=B_SPLINE_SURFACE_WITH_KNOTS('',3,3,((#99552,#99553,#99554,#99555),
(#99556,#99557,#99558,#99559),(#99560,#99561,#99562,#99563),(#99564,#99565,
#99566,#99567),(#99568,#99569,#99570,#99571)),.UNSPECIFIED.,.F.,.F.,.F.,
(4,1,4),(4,4),(0.,0.5,1.),(0.,0.324683822128098),.UNSPECIFIED.);
#18957=B_SPLINE_SURFACE_WITH_KNOTS('',3,3,((#99578,#99579,#99580,#99581),
(#99582,#99583,#99584,#99585),(#99586,#99587,#99588,#99589),(#99590,#99591,
#99592,#99593),(#99594,#99595,#99596,#99597)),.UNSPECIFIED.,.F.,.F.,.F.,
(4,1,4),(4,4),(-4.017133134979E-5,0.5,1.),(-4.01713313514047E-5,0.0546115211509732),
 .UNSPECIFIED.);
#18958=B_SPLINE_SURFACE_WITH_KNOTS('',3,3,((#99598,#99599,#99600,#99601),
(#99602,#99603,#99604,#99605),(#99606,#99607,#99608,#99609),(#99610,#99611,
#99612,#99613),(#99614,#99615,#99616,#99617)),.UNSPECIFIED.,.F.,.F.,.F.,
(4,1,4),(4,4),(-4.89933240230808E-5,0.309230284442265,0.721537330365286),
(-4.89933240233201E-5,0.0862352312335747),.UNSPECIFIED.);
#18959=B_SPLINE_SURFACE_WITH_KNOTS('',3,3,((#99619,#99620,#99621,#99622),
(#99623,#99624,#99625,#99626),(#99627,#99628,#99629,#99630),(#99631,#99632,
#99633,#99634)),.UNSPECIFIED.,.F.,.F.,.F.,(4,4),(4,4),(0.640913278953462,
1.),(-1.2330723644364E-15,0.0441554944100176),.UNSPECIFIED.);
#19973=ADVANCED_FACE('',(#6039),#4980,.T.);
#19974=ADVANCED_FACE('',(#6040),#4981,.T.);
#19975=ADVANCED_FACE('',(#6041),#4982,.T.);
#19976=ADVANCED_FACE('',(#6042),#4983,.T.);
#19977=ADVANCED_FACE('',(#6043),#217,.T.);
#19978=ADVANCED_FACE('',(#6044),#218,.T.);
#19979=ADVANCED_FACE('',(#6045),#219,.T.);
#19980=ADVANCED_FACE('',(#6046),#220,.T.);
#19981=ADVANCED_FACE('',(#6047),#4984,.T.);
#19982=ADVANCED_FACE('',(#6048),#1652,.T.);
#19983=ADVANCED_FACE('',(#6049),#4985,.T.);
#19984=ADVANCED_FACE('',(#6050,#1782,#1783),#1653,.T.);
#19985=ADVANCED_FACE('',(#6051),#1654,.T.);
#19986=ADVANCED_FACE('',(#6052),#4986,.T.);
#19987=ADVANCED_FACE('',(#6053),#4987,.T.);
#19988=ADVANCED_FACE('',(#6054),#221,.T.);
#19989=ADVANCED_FACE('',(#6055),#4988,.T.);
#19990=ADVANCED_FACE('',(#6056),#222,.T.);
#19991=ADVANCED_FACE('',(#6057),#18938,.F.);
#19992=ADVANCED_FACE('',(#6058),#18939,.T.);
#19993=ADVANCED_FACE('',(#6059),#18940,.F.);
#19994=ADVANCED_FACE('',(#6060,#1784,#1785),#1655,.T.);
#19995=ADVANCED_FACE('',(#6061),#4989,.T.);
#19996=ADVANCED_FACE('',(#6062),#223,.T.);
#19997=ADVANCED_FACE('',(#6063),#224,.T.);
#19998=ADVANCED_FACE('',(#6064),#18941,.F.);
#19999=ADVANCED_FACE('',(#6065),#18942,.T.);
#20000=ADVANCED_FACE('',(#6066),#18943,.F.);
#20001=ADVANCED_FACE('',(#6067),#18944,.F.);
#20002=ADVANCED_FACE('',(#6068),#18945,.F.);
#20003=ADVANCED_FACE('',(#6069),#18946,.F.);
#20004=ADVANCED_FACE('',(#6070),#18947,.F.);
#20005=ADVANCED_FACE('',(#6071),#4990,.T.);
#20006=ADVANCED_FACE('',(#6072),#1282,.T.);
#20007=ADVANCED_FACE('',(#6073),#4991,.T.);
#20008=ADVANCED_FACE('',(#6074),#18948,.F.);
#20009=ADVANCED_FACE('',(#6075),#18949,.F.);
#20010=ADVANCED_FACE('',(#6076),#18950,.F.);
#20011=ADVANCED_FACE('',(#6077),#18951,.F.);
#20012=ADVANCED_FACE('',(#6078),#1656,.T.);
#20013=ADVANCED_FACE('',(#6079),#4992,.T.);
#20014=ADVANCED_FACE('',(#6080),#1657,.T.);
#20015=ADVANCED_FACE('',(#6081),#1658,.T.);
#20016=ADVANCED_FACE('',(#6082),#18952,.F.);
#20017=ADVANCED_FACE('',(#6083),#18953,.F.);
#20018=ADVANCED_FACE('',(#6084),#18954,.F.);
#20019=ADVANCED_FACE('',(#6085),#18955,.F.);
#20020=ADVANCED_FACE('',(#6086),#4993,.T.);
#20021=ADVANCED_FACE('',(#6087),#18956,.F.);
#20022=ADVANCED_FACE('',(#6088),#18957,.F.);
#20023=ADVANCED_FACE('',(#6089),#18958,.F.);
#20024=ADVANCED_FACE('',(#6090),#18959,.F.);
#20025=ADVANCED_FACE('',(#6091),#4994,.F.);
#20026=ADVANCED_FACE('',(#6092,#1786,#1787),#1659,.T.);
#20027=ADVANCED_FACE('',(#6093),#1283,.T.);
#20028=ADVANCED_FACE('',(#6094),#4995,.F.);
#20029=ADVANCED_FACE('',(#6095),#1284,.T.);
#20030=ADVANCED_FACE('',(#6096),#1285,.T.);
#20031=ADVANCED_FACE('',(#6097),#4996,.F.);
#20032=ADVANCED_FACE('',(#6098),#1286,.T.);
#20033=ADVANCED_FACE('',(#6099,#1788,#1789),#1660,.T.);
#20034=ADVANCED_FACE('',(#6100),#1287,.T.);
#20035=ADVANCED_FACE('',(#6101),#4997,.F.);
#20036=ADVANCED_FACE('',(#6102),#1288,.T.);
#20037=ADVANCED_FACE('',(#6103),#1289,.T.);
#20038=ADVANCED_FACE('',(#6104),#4998,.F.);
#20039=ADVANCED_FACE('',(#6105),#1290,.T.);
#20040=ADVANCED_FACE('',(#6106),#1661,.T.);
#20041=ADVANCED_FACE('',(#6107),#4999,.T.);
#20042=ADVANCED_FACE('',(#6108),#5000,.F.);
#20043=ADVANCED_FACE('',(#6109),#1662,.T.);
#20126=CLOSED_SHELL('',(#19973,#19974,#19975,#19976,#19977,#19978,#19979,
#19980,#19981,#19982,#19983,#19984,#19985,#19986,#19987,#19988,#19989,#19990,
#19991,#19992,#19993,#19994,#19995,#19996,#19997,#19998,#19999,#20000,#20001,
#20002,#20003,#20004,#20005,#20006,#20007,#20008,#20009,#20010,#20011,#20012,
#20013,#20014,#20015,#20016,#20017,#20018,#20019,#20020,#20021,#20022,#20023,
#20024,#20025,#20026,#20027,#20028,#20029,#20030,#20031,#20032,#20033,#20034,
#20035,#20036,#20037,#20038,#20039,#20040,#20041,#20042,#20043));
#22218=AXIS2_PLACEMENT_3D('',#97801,#27496,#27497);
#22219=AXIS2_PLACEMENT_3D('',#97802,#27498,#27499);
#22220=AXIS2_PLACEMENT_3D('',#97805,#27500,#27501);
#22221=AXIS2_PLACEMENT_3D('',#97809,#27503,#27504);
#22222=AXIS2_PLACEMENT_3D('',#97811,#27506,#27507);
#22223=AXIS2_PLACEMENT_3D('',#97814,#27508,#27509);
#22224=AXIS2_PLACEMENT_3D('',#97817,#27511,#27512);
#22225=AXIS2_PLACEMENT_3D('',#97819,#27514,#27515);
#22226=AXIS2_PLACEMENT_3D('',#97821,#27516,#27517);
#22227=AXIS2_PLACEMENT_3D('',#97825,#27519,#27520);
#22228=AXIS2_PLACEMENT_3D('',#97827,#27522,#27523);
#22229=AXIS2_PLACEMENT_3D('',#97829,#27524,#27525);
#22230=AXIS2_PLACEMENT_3D('',#97832,#27527,#27528);
#22231=AXIS2_PLACEMENT_3D('',#97834,#27530,#27531);
#22232=AXIS2_PLACEMENT_3D('',#97835,#27532,#27533);
#22233=AXIS2_PLACEMENT_3D('',#97836,#27534,#27535);
#22234=AXIS2_PLACEMENT_3D('',#97837,#27536,#27537);
#22235=AXIS2_PLACEMENT_3D('',#97838,#27538,#27539);
#22236=AXIS2_PLACEMENT_3D('',#97839,#27540,#27541);
#22237=AXIS2_PLACEMENT_3D('',#97840,#27542,#27543);
#22238=AXIS2_PLACEMENT_3D('',#97841,#27544,#27545);
#22239=AXIS2_PLACEMENT_3D('',#97842,#27546,#27547);
#22240=AXIS2_PLACEMENT_3D('',#97846,#27549,#27550);
#22241=AXIS2_PLACEMENT_3D('',#97848,#27552,#27553);
#22242=AXIS2_PLACEMENT_3D('',#97852,#27556,#27557);
#22243=AXIS2_PLACEMENT_3D('',#97855,#27559,#27560);
#22244=AXIS2_PLACEMENT_3D('',#97856,#27561,#27562);
#22245=AXIS2_PLACEMENT_3D('',#97917,#27565,#27566);
#22246=AXIS2_PLACEMENT_3D('',#97919,#27567,#27568);
#22247=AXIS2_PLACEMENT_3D('',#97920,#27569,#27570);
#22248=AXIS2_PLACEMENT_3D('',#97921,#27571,#27572);
#22249=AXIS2_PLACEMENT_3D('',#97924,#27574,#27575);
#22250=AXIS2_PLACEMENT_3D('',#97925,#27576,#27577);
#22251=AXIS2_PLACEMENT_3D('',#97927,#27578,#27579);
#22252=AXIS2_PLACEMENT_3D('',#97931,#27581,#27582);
#22253=AXIS2_PLACEMENT_3D('',#97933,#27584,#27585);
#22254=AXIS2_PLACEMENT_3D('',#97934,#27586,#27587);
#22255=AXIS2_PLACEMENT_3D('',#97935,#27588,#27589);
#22256=AXIS2_PLACEMENT_3D('',#97938,#27591,#27592);
#22257=AXIS2_PLACEMENT_3D('',#97940,#27594,#27595);
#22258=AXIS2_PLACEMENT_3D('',#97941,#27596,#27597);
#22259=AXIS2_PLACEMENT_3D('',#98111,#27598,#27599);
#22260=AXIS2_PLACEMENT_3D('',#98311,#27600,#27601);
#22261=AXIS2_PLACEMENT_3D('',#98514,#27603,#27604);
#22262=AXIS2_PLACEMENT_3D('',#98515,#27605,#27606);
#22263=AXIS2_PLACEMENT_3D('',#98548,#27608,#27609);
#22264=AXIS2_PLACEMENT_3D('',#98550,#27610,#27611);
#22265=AXIS2_PLACEMENT_3D('',#98551,#27612,#27613);
#22266=AXIS2_PLACEMENT_3D('',#98553,#27614,#27615);
#22267=AXIS2_PLACEMENT_3D('',#98556,#27617,#27618);
#22268=AXIS2_PLACEMENT_3D('',#98557,#27619,#27620);
#22269=AXIS2_PLACEMENT_3D('',#98558,#27621,#27622);
#22270=AXIS2_PLACEMENT_3D('',#98559,#27623,#27624);
#22271=AXIS2_PLACEMENT_3D('',#98560,#27625,#27626);
#22272=AXIS2_PLACEMENT_3D('',#98736,#27627,#27628);
#22273=AXIS2_PLACEMENT_3D('',#98954,#27630,#27631);
#22274=AXIS2_PLACEMENT_3D('',#99114,#27632,#27633);
#22275=AXIS2_PLACEMENT_3D('',#99140,#27634,#27635);
#22276=AXIS2_PLACEMENT_3D('',#99162,#27636,#27637);
#22277=AXIS2_PLACEMENT_3D('',#99192,#27638,#27639);
#22278=AXIS2_PLACEMENT_3D('',#99246,#27640,#27641);
#22279=AXIS2_PLACEMENT_3D('',#99250,#27643,#27644);
#22280=AXIS2_PLACEMENT_3D('',#99252,#27646,#27647);
#22281=AXIS2_PLACEMENT_3D('',#99255,#27648,#27649);
#22282=AXIS2_PLACEMENT_3D('',#99256,#27650,#27651);
#22283=AXIS2_PLACEMENT_3D('',#99257,#27652,#27653);
#22284=AXIS2_PLACEMENT_3D('',#99258,#27654,#27655);
#22285=AXIS2_PLACEMENT_3D('',#99299,#27658,#27659);
#22286=AXIS2_PLACEMENT_3D('',#99305,#27660,#27661);
#22287=AXIS2_PLACEMENT_3D('',#99363,#27662,#27663);
#22288=AXIS2_PLACEMENT_3D('',#99392,#27664,#27665);
#22289=AXIS2_PLACEMENT_3D('',#99398,#27668,#27669);
#22290=AXIS2_PLACEMENT_3D('',#99402,#27671,#27672);
#22291=AXIS2_PLACEMENT_3D('',#99424,#27673,#27674);
#22292=AXIS2_PLACEMENT_3D('',#99427,#27676,#27677);
#22293=AXIS2_PLACEMENT_3D('',#99428,#27678,#27679);
#22294=AXIS2_PLACEMENT_3D('',#99450,#27680,#27681);
#22295=AXIS2_PLACEMENT_3D('',#99454,#27683,#27684);
#22296=AXIS2_PLACEMENT_3D('',#99456,#27686,#27687);
#22297=AXIS2_PLACEMENT_3D('',#99477,#27688,#27689);
#22298=AXIS2_PLACEMENT_3D('',#99479,#27690,#27691);
#22299=AXIS2_PLACEMENT_3D('',#99504,#27692,#27693);
#22300=AXIS2_PLACEMENT_3D('',#99545,#27694,#27695);
#22301=AXIS2_PLACEMENT_3D('',#99576,#27697,#27698);
#22302=AXIS2_PLACEMENT_3D('',#99577,#27699,#27700);
#22303=AXIS2_PLACEMENT_3D('',#99618,#27701,#27702);
#22304=AXIS2_PLACEMENT_3D('',#99635,#27703,#27704);
#22305=AXIS2_PLACEMENT_3D('',#99638,#27707,#27708);
#22306=AXIS2_PLACEMENT_3D('',#99640,#27709,#27710);
#22307=AXIS2_PLACEMENT_3D('',#99642,#27711,#27712);
#22308=AXIS2_PLACEMENT_3D('',#99643,#27713,#27714);
#22309=AXIS2_PLACEMENT_3D('',#99645,#27715,#27716);
#22310=AXIS2_PLACEMENT_3D('',#99647,#27717,#27718);
#22311=AXIS2_PLACEMENT_3D('',#99648,#27719,#27720);
#22312=AXIS2_PLACEMENT_3D('',#99649,#27721,#27722);
#22313=AXIS2_PLACEMENT_3D('',#99653,#27724,#27725);
#22314=AXIS2_PLACEMENT_3D('',#99654,#27726,#27727);
#22315=AXIS2_PLACEMENT_3D('',#99655,#27728,#27729);
#22316=AXIS2_PLACEMENT_3D('',#99656,#27730,#27731);
#22317=AXIS2_PLACEMENT_3D('',#99657,#27732,#27733);
#22318=AXIS2_PLACEMENT_3D('',#99659,#27734,#27735);
#22319=AXIS2_PLACEMENT_3D('',#99661,#27736,#27737);
#22320=AXIS2_PLACEMENT_3D('',#99662,#27738,#27739);
#22321=AXIS2_PLACEMENT_3D('',#99663,#27740,#27741);
#22322=AXIS2_PLACEMENT_3D('',#99667,#27743,#27744);
#22323=AXIS2_PLACEMENT_3D('',#99668,#27745,#27746);
#22324=AXIS2_PLACEMENT_3D('',#99669,#27747,#27748);
#22325=AXIS2_PLACEMENT_3D('',#99671,#27749,#27750);
#22326=AXIS2_PLACEMENT_3D('',#99672,#27751,#27752);
#22327=AXIS2_PLACEMENT_3D('',#99673,#27753,#27754);
#22328=AXIS2_PLACEMENT_3D('',#99676,#27756,#27757);
#22329=AXIS2_PLACEMENT_3D('',#99677,#27758,#27759);
#22330=AXIS2_PLACEMENT_3D('',#99679,#27760,#27761);
#22331=AXIS2_PLACEMENT_3D('',#99681,#27762,#27763);
#22332=AXIS2_PLACEMENT_3D('',#99682,#27764,#27765);
#22333=AXIS2_PLACEMENT_3D('',#99683,#27766,#27767);
#22334=AXIS2_PLACEMENT_3D('',#99687,#27769,#27770);
#22335=AXIS2_PLACEMENT_3D('',#99688,#27771,#27772);
#22336=AXIS2_PLACEMENT_3D('',#99689,#27773,#27774);
#22337=AXIS2_PLACEMENT_3D('',#99690,#27775,#27776);
#22338=AXIS2_PLACEMENT_3D('',#99691,#27777,#27778);
#22339=AXIS2_PLACEMENT_3D('',#99693,#27779,#27780);
#22340=AXIS2_PLACEMENT_3D('',#99695,#27781,#27782);
#22341=AXIS2_PLACEMENT_3D('',#99696,#27783,#27784);
#22342=AXIS2_PLACEMENT_3D('',#99697,#27785,#27786);
#22343=AXIS2_PLACEMENT_3D('',#99701,#27788,#27789);
#22344=AXIS2_PLACEMENT_3D('',#99702,#27790,#27791);
#22345=AXIS2_PLACEMENT_3D('',#99703,#27792,#27793);
#22346=AXIS2_PLACEMENT_3D('',#99704,#27794,#27795);
#22347=AXIS2_PLACEMENT_3D('',#99705,#27796,#27797);
#22348=AXIS2_PLACEMENT_3D('',#99706,#27798,#27799);
#22349=AXIS2_PLACEMENT_3D('',#99708,#27801,#27802);
#22350=AXIS2_PLACEMENT_3D('',#99710,#27804,#27805);
#27496=DIRECTION('axis',(0.,0.,1.));
#27497=DIRECTION('refdir',(1.,0.,0.));
#27498=DIRECTION('center_axis',(0.,-1.,0.));
#27499=DIRECTION('ref_axis',(0.707106781186558,0.,0.707106781186537));
#27500=DIRECTION('center_axis',(0.,-1.,0.));
#27501=DIRECTION('ref_axis',(1.,0.,0.));
#27502=DIRECTION('',(0.,-1.,0.));
#27503=DIRECTION('center_axis',(0.,1.,0.));
#27504=DIRECTION('ref_axis',(0.,0.,1.));
#27505=DIRECTION('',(0.,1.,0.));
#27506=DIRECTION('center_axis',(1.,0.,0.));
#27507=DIRECTION('ref_axis',(0.,-0.707106781186534,0.707106781186561));
#27508=DIRECTION('center_axis',(1.,0.,0.));
#27509=DIRECTION('ref_axis',(0.,0.,1.));
#27510=DIRECTION('',(1.,0.,0.));
#27511=DIRECTION('center_axis',(-1.,0.,0.));
#27512=DIRECTION('ref_axis',(0.,-1.,0.));
#27513=DIRECTION('',(-1.,0.,0.));
#27514=DIRECTION('center_axis',(0.,1.,0.));
#27515=DIRECTION('ref_axis',(-0.707106781186558,0.,0.707106781186537));
#27516=DIRECTION('center_axis',(0.,1.,0.));
#27517=DIRECTION('ref_axis',(-1.,0.,0.));
#27518=DIRECTION('',(0.,1.,0.));
#27519=DIRECTION('center_axis',(0.,-1.,0.));
#27520=DIRECTION('ref_axis',(0.,0.,1.));
#27521=DIRECTION('',(0.,-1.,0.));
#27522=DIRECTION('center_axis',(-1.,0.,0.));
#27523=DIRECTION('ref_axis',(0.,0.707106781186555,0.70710678118654));
#27524=DIRECTION('center_axis',(-1.,0.,0.));
#27525=DIRECTION('ref_axis',(0.,0.,1.));
#27526=DIRECTION('',(-1.,0.,0.));
#27527=DIRECTION('center_axis',(1.,0.,0.));
#27528=DIRECTION('ref_axis',(0.,1.,0.));
#27529=DIRECTION('',(1.,0.,0.));
#27530=DIRECTION('center_axis',(-0.40824829046386,-0.816496580927729,0.40824829046386));
#27531=DIRECTION('ref_axis',(-0.57735026918963,0.577350269189623,0.577350269189624));
#27532=DIRECTION('center_axis',(0.,0.,1.));
#27533=DIRECTION('ref_axis',(-0.707106781186551,0.707106781186544,0.));
#27534=DIRECTION('center_axis',(-0.408248290463851,-0.408248290463851,-0.816496580927738));
#27535=DIRECTION('ref_axis',(-0.577350269189626,-0.577350269189631,0.57735026918962));
#27536=DIRECTION('center_axis',(0.,0.,1.));
#27537=DIRECTION('ref_axis',(-0.70710678118655,-0.707106781186544,0.));
#27538=DIRECTION('center_axis',(-0.408248290463842,-0.816496580927738,-0.40824829046386));
#27539=DIRECTION('ref_axis',(0.577350269189618,-0.577350269189612,0.577350269189648));
#27540=DIRECTION('center_axis',(0.,0.,1.));
#27541=DIRECTION('ref_axis',(0.70710678118655,-0.707106781186544,0.));
#27542=DIRECTION('center_axis',(0.40824829046386,-0.816496580927729,0.40824829046386));
#27543=DIRECTION('ref_axis',(0.57735026918963,0.577350269189623,0.577350269189624));
#27544=DIRECTION('center_axis',(0.,0.,1.));
#27545=DIRECTION('ref_axis',(0.707106781186551,0.707106781186544,0.));
#27546=DIRECTION('center_axis',(0.,0.,1.));
#27547=DIRECTION('ref_axis',(-0.70710678118655,-0.707106781186545,0.));
#27548=DIRECTION('',(0.,0.,-1.));
#27549=DIRECTION('center_axis',(0.,0.,1.));
#27550=DIRECTION('ref_axis',(-1.,0.,0.));
#27551=DIRECTION('',(0.,0.,1.));
#27552=DIRECTION('center_axis',(-1.,0.,0.));
#27553=DIRECTION('ref_axis',(0.,0.,1.));
#27554=DIRECTION('',(0.,0.,1.));
#27555=DIRECTION('',(0.,1.,0.));
#27556=DIRECTION('center_axis',(0.,0.,-1.));
#27557=DIRECTION('ref_axis',(-0.707106781186551,0.707106781186544,0.));
#27558=DIRECTION('',(0.,0.,-1.));
#27559=DIRECTION('center_axis',(0.,0.,1.));
#27560=DIRECTION('ref_axis',(1.48029736616688E-14,1.,0.));
#27561=DIRECTION('center_axis',(0.,1.,0.));
#27562=DIRECTION('ref_axis',(0.,0.,1.));
#27563=DIRECTION('',(0.,0.,1.));
#27564=DIRECTION('',(1.,0.,0.));
#27565=DIRECTION('center_axis',(0.,1.,0.));
#27566=DIRECTION('ref_axis',(1.,0.,0.));
#27567=DIRECTION('center_axis',(0.,1.,0.));
#27568=DIRECTION('ref_axis',(1.,0.,0.));
#27569=DIRECTION('center_axis',(0.,0.,1.));
#27570=DIRECTION('ref_axis',(0.,-1.,0.));
#27571=DIRECTION('center_axis',(0.,0.,1.));
#27572=DIRECTION('ref_axis',(0.707106781186551,0.707106781186544,0.));
#27573=DIRECTION('',(0.,0.,-1.));
#27574=DIRECTION('center_axis',(0.,0.,1.));
#27575=DIRECTION('ref_axis',(1.,0.,0.));
#27576=DIRECTION('center_axis',(0.,1.,0.));
#27577=DIRECTION('ref_axis',(0.99894638116538,0.,-0.0458925653738368));
#27578=DIRECTION('center_axis',(0.,-1.,0.));
#27579=DIRECTION('ref_axis',(0.995787744886652,0.,-0.091688424206963));
#27580=DIRECTION('',(0.,-1.,0.));
#27581=DIRECTION('center_axis',(0.,1.,0.));
#27582=DIRECTION('ref_axis',(1.,0.,0.));
#27583=DIRECTION('',(0.,1.,0.));
#27584=DIRECTION('center_axis',(0.,0.,1.));
#27585=DIRECTION('ref_axis',(1.,0.,0.));
#27586=DIRECTION('center_axis',(0.0916884242070712,0.,0.995787744886642));
#27587=DIRECTION('ref_axis',(2.70308839529112E-15,1.,-2.48890304916212E-16));
#27588=DIRECTION('center_axis',(0.,0.,-1.));
#27589=DIRECTION('ref_axis',(0.70710678118655,-0.707106781186545,0.));
#27590=DIRECTION('',(0.,0.,-1.));
#27591=DIRECTION('center_axis',(0.,0.,1.));
#27592=DIRECTION('ref_axis',(-1.48029736616688E-14,-1.,0.));
#27593=DIRECTION('',(0.,0.,1.));
#27594=DIRECTION('center_axis',(0.,0.,1.));
#27595=DIRECTION('ref_axis',(1.,0.,0.));
#27596=DIRECTION('center_axis',(0.0916884242070274,0.,0.995787744886646));
#27597=DIRECTION('ref_axis',(1.35154419764492E-14,-1.,-1.24445152457987E-15));
#27598=DIRECTION('center_axis',(-0.342464185150441,0.,-0.939530883946475));
#27599=DIRECTION('ref_axis',(0.,1.,0.));
#27600=DIRECTION('center_axis',(0.,1.,0.));
#27601=DIRECTION('ref_axis',(-0.991776726791891,0.,0.127980171096785));
#27602=DIRECTION('',(0.,1.,0.));
#27603=DIRECTION('center_axis',(-0.341922938227805,0.,-0.939727994854716));
#27604=DIRECTION('ref_axis',(0.939727994854716,0.,-0.341922938227805));
#27605=DIRECTION('center_axis',(0.,-1.,0.));
#27606=DIRECTION('ref_axis',(0.,0.,-1.));
#27607=DIRECTION('',(-1.,0.,0.));
#27608=DIRECTION('center_axis',(0.,-1.,0.));
#27609=DIRECTION('ref_axis',(1.,0.,0.));
#27610=DIRECTION('center_axis',(0.,-1.,0.));
#27611=DIRECTION('ref_axis',(1.,0.,0.));
#27612=DIRECTION('center_axis',(0.,1.,0.));
#27613=DIRECTION('ref_axis',(-0.9989463811658,0.,-0.0458925653646838));
#27614=DIRECTION('center_axis',(0.,-1.,4.03621661973593E-14));
#27615=DIRECTION('ref_axis',(-1.,0.,0.));
#27616=DIRECTION('',(0.,-1.,0.));
#27617=DIRECTION('center_axis',(0.,1.,7.06337908453787E-14));
#27618=DIRECTION('ref_axis',(-0.995787744888473,6.47630097698012E-15,-0.0916884241871869));
#27619=DIRECTION('center_axis',(0.,0.,1.));
#27620=DIRECTION('ref_axis',(1.,0.,0.));
#27621=DIRECTION('center_axis',(-0.0916884241872355,0.,0.995787744888469));
#27622=DIRECTION('ref_axis',(-2.70308839471129E-15,1.,-2.48890304808522E-16));
#27623=DIRECTION('center_axis',(0.,0.,1.));
#27624=DIRECTION('ref_axis',(1.,0.,0.));
#27625=DIRECTION('center_axis',(-0.0916884241872959,0.,0.995787744888463));
#27626=DIRECTION('ref_axis',(-1.54000185901395E-15,-1.,-1.4179763149657E-16));
#27627=DIRECTION('center_axis',(0.341922938227109,6.95538437848544E-15,
-0.939727994854969));
#27628=DIRECTION('ref_axis',(-9.06088119400516E-31,-1.,-7.40148683083437E-15));
#27629=DIRECTION('',(0.,1.,0.));
#27630=DIRECTION('center_axis',(0.,1.,0.));
#27631=DIRECTION('ref_axis',(0.99622596754828,0.,0.0867975897274464));
#27632=DIRECTION('center_axis',(-0.342464185149375,0.,0.939530883946863));
#27633=DIRECTION('ref_axis',(0.,1.,0.));
#27634=DIRECTION('center_axis',(-0.290611853669958,-0.507124729938608,0.811399567901786));
#27635=DIRECTION('ref_axis',(2.95685193295205E-17,0.847998304005092,0.529998940003174));
#27636=DIRECTION('center_axis',(-0.169633066553524,-0.522317820164791,0.835708512263665));
#27637=DIRECTION('ref_axis',(-4.86759141432297E-17,0.847998304005088,0.52999894000318));
#27638=DIRECTION('center_axis',(-0.157204875383854,3.6547284145087E-15,
0.987566011543303));
#27639=DIRECTION('ref_axis',(7.52525386954664E-31,1.,-3.7007434154172E-15));
#27640=DIRECTION('center_axis',(0.,0.,-1.));
#27641=DIRECTION('ref_axis',(-0.707106781186547,0.707106781186547,0.));
#27642=DIRECTION('',(0.,0.,-1.));
#27643=DIRECTION('center_axis',(0.,0.,1.));
#27644=DIRECTION('ref_axis',(0.,1.,0.));
#27645=DIRECTION('',(0.,0.,1.));
#27646=DIRECTION('center_axis',(0.,-1.,0.));
#27647=DIRECTION('ref_axis',(0.,0.,-1.));
#27648=DIRECTION('center_axis',(7.40148683083437E-15,0.,-1.));
#27649=DIRECTION('ref_axis',(0.,1.,0.));
#27650=DIRECTION('center_axis',(0.,1.,0.));
#27651=DIRECTION('ref_axis',(1.5559876576226E-16,0.,-1.));
#27652=DIRECTION('center_axis',(0.,-1.,0.));
#27653=DIRECTION('ref_axis',(1.5559876576226E-16,0.,-1.));
#27654=DIRECTION('center_axis',(0.,0.,1.));
#27655=DIRECTION('ref_axis',(0.707106781186547,0.707106781186547,0.));
#27656=DIRECTION('',(0.,0.,-1.));
#27657=DIRECTION('',(0.,0.,1.));
#27658=DIRECTION('center_axis',(0.15720487538553,0.,0.987566011543036));
#27659=DIRECTION('ref_axis',(0.987566011543036,0.,-0.15720487538553));
#27660=DIRECTION('center_axis',(-0.169633066555186,0.522317820164643,-0.835708512263421));
#27661=DIRECTION('ref_axis',(1.0172704914008E-16,0.847998304005086,0.529998940003184));
#27662=DIRECTION('center_axis',(-0.290611853669808,0.507124729938623,-0.81139956790183));
#27663=DIRECTION('ref_axis',(1.15214297628471E-16,0.847998304005098,0.529998940003164));
#27664=DIRECTION('center_axis',(-1.,0.,0.));
#27665=DIRECTION('ref_axis',(0.,0.,1.));
#27666=DIRECTION('',(0.,1.,0.));
#27667=DIRECTION('',(0.,0.,1.));
#27668=DIRECTION('center_axis',(1.,0.,0.));
#27669=DIRECTION('ref_axis',(0.,0.961248746164355,0.275682513042551));
#27670=DIRECTION('',(0.,-0.52999894000318,0.847998304005088));
#27671=DIRECTION('center_axis',(1.,0.,0.));
#27672=DIRECTION('ref_axis',(0.,-0.63620934106487,0.771516477038439));
#27673=DIRECTION('center_axis',(0.,1.,0.));
#27674=DIRECTION('ref_axis',(1.,0.,3.16411030729924E-16));
#27675=DIRECTION('',(0.,1.,0.));
#27676=DIRECTION('center_axis',(0.,1.,0.));
#27677=DIRECTION('ref_axis',(1.,0.,3.16411030729924E-16));
#27678=DIRECTION('center_axis',(1.,0.,0.));
#27679=DIRECTION('ref_axis',(0.,0.,-1.));
#27680=DIRECTION('center_axis',(-1.,0.,0.));
#27681=DIRECTION('ref_axis',(0.,0.6339690029848,-0.773358457155838));
#27682=DIRECTION('',(0.,0.52999894000318,-0.847998304005088));
#27683=DIRECTION('center_axis',(-1.,0.,0.));
#27684=DIRECTION('ref_axis',(0.,0.961248746164355,0.275682513042551));
#27685=DIRECTION('',(0.,0.,-1.));
#27686=DIRECTION('center_axis',(1.,0.,0.));
#27687=DIRECTION('ref_axis',(0.,0.,-1.));
#27688=DIRECTION('center_axis',(0.169039506365408,-0.52237187163154,0.835794994610462));
#27689=DIRECTION('ref_axis',(6.12619120378935E-17,-0.847998304005087,-0.529998940003181));
#27690=DIRECTION('center_axis',(-0.290495237999518,0.507143497604778,-0.81142959616765));
#27691=DIRECTION('ref_axis',(0.941484765039641,1.58293525692317E-16,-0.337055540227797));
#27692=DIRECTION('center_axis',(0.127825287380035,0.,0.991796700895003));
#27693=DIRECTION('ref_axis',(0.,-1.,0.));
#27694=DIRECTION('center_axis',(1.,0.,0.));
#27695=DIRECTION('ref_axis',(0.,-0.961248746164355,-0.275682513042551));
#27696=DIRECTION('',(1.,0.,0.));
#27697=DIRECTION('center_axis',(0.290495237999669,0.507143497604755,-0.811429596167611));
#27698=DIRECTION('ref_axis',(-9.8030109697363E-17,-0.847998304005089,-0.529998940003178));
#27699=DIRECTION('center_axis',(-0.169039506363714,-0.522371871631687,0.835794994610712));
#27700=DIRECTION('ref_axis',(-0.980154284762346,-2.33134209272865E-16,-0.198236167391356));
#27701=DIRECTION('center_axis',(-0.127825287380379,-3.67038511026951E-15,
0.991796700894958));
#27702=DIRECTION('ref_axis',(-0.991796700894958,2.7885015020519E-32,-0.127825287380379));
#27703=DIRECTION('center_axis',(1.,0.,0.));
#27704=DIRECTION('ref_axis',(0.,0.961248746164355,0.275682513042551));
#27705=DIRECTION('',(-1.,0.,0.));
#27706=DIRECTION('',(1.,0.,0.));
#27707=DIRECTION('center_axis',(0.,-1.,0.));
#27708=DIRECTION('ref_axis',(0.,0.,-1.));
#27709=DIRECTION('center_axis',(0.,-1.,0.));
#27710=DIRECTION('ref_axis',(1.,0.,0.));
#27711=DIRECTION('center_axis',(0.,-1.,0.));
#27712=DIRECTION('ref_axis',(1.,0.,0.));
#27713=DIRECTION('center_axis',(0.,1.,0.));
#27714=DIRECTION('ref_axis',(0.,0.,1.));
#27715=DIRECTION('center_axis',(-1.,0.,0.));
#27716=DIRECTION('ref_axis',(0.,0.,-1.));
#27717=DIRECTION('center_axis',(0.,1.,0.));
#27718=DIRECTION('ref_axis',(1.,0.,0.));
#27719=DIRECTION('center_axis',(0.,1.,0.));
#27720=DIRECTION('ref_axis',(1.,0.,0.));
#27721=DIRECTION('center_axis',(0.,1.,0.));
#27722=DIRECTION('ref_axis',(1.,0.,0.));
#27723=DIRECTION('',(0.,1.,0.));
#27724=DIRECTION('center_axis',(0.,-1.,0.));
#27725=DIRECTION('ref_axis',(1.,0.,0.));
#27726=DIRECTION('center_axis',(0.,-1.,0.));
#27727=DIRECTION('ref_axis',(1.,0.,0.));
#27728=DIRECTION('center_axis',(0.,-1.,0.));
#27729=DIRECTION('ref_axis',(0.,0.,-1.));
#27730=DIRECTION('center_axis',(-1.,0.,0.));
#27731=DIRECTION('ref_axis',(0.,0.,1.));
#27732=DIRECTION('center_axis',(0.,1.,0.));
#27733=DIRECTION('ref_axis',(0.,0.,1.));
#27734=DIRECTION('center_axis',(-1.,0.,1.22464679914735E-16));
#27735=DIRECTION('ref_axis',(-1.22464679914735E-16,0.,-1.));
#27736=DIRECTION('center_axis',(0.,1.,0.));
#27737=DIRECTION('ref_axis',(1.,0.,0.));
#27738=DIRECTION('center_axis',(0.,1.,0.));
#27739=DIRECTION('ref_axis',(1.,0.,0.));
#27740=DIRECTION('center_axis',(0.,1.,0.));
#27741=DIRECTION('ref_axis',(1.,0.,0.));
#27742=DIRECTION('',(0.,1.,0.));
#27743=DIRECTION('center_axis',(0.,-1.,0.));
#27744=DIRECTION('ref_axis',(1.,0.,0.));
#27745=DIRECTION('center_axis',(0.,-1.,0.));
#27746=DIRECTION('ref_axis',(1.,0.,0.));
#27747=DIRECTION('center_axis',(0.,-1.,0.));
#27748=DIRECTION('ref_axis',(0.,0.,-1.));
#27749=DIRECTION('center_axis',(0.,1.,0.));
#27750=DIRECTION('ref_axis',(1.,0.,0.));
#27751=DIRECTION('center_axis',(-1.,0.,-1.22464679914735E-16));
#27752=DIRECTION('ref_axis',(-1.22464679914735E-16,0.,1.));
#27753=DIRECTION('center_axis',(0.,1.,0.));
#27754=DIRECTION('ref_axis',(0.,0.,1.));
#27755=DIRECTION('',(-1.,0.,0.));
#27756=DIRECTION('center_axis',(0.,1.,0.));
#27757=DIRECTION('ref_axis',(1.,0.,0.));
#27758=DIRECTION('center_axis',(0.,1.,0.));
#27759=DIRECTION('ref_axis',(0.,0.,1.));
#27760=DIRECTION('center_axis',(-1.,0.,0.));
#27761=DIRECTION('ref_axis',(0.,0.,-1.));
#27762=DIRECTION('center_axis',(0.,1.,0.));
#27763=DIRECTION('ref_axis',(1.,0.,0.));
#27764=DIRECTION('center_axis',(0.,1.,0.));
#27765=DIRECTION('ref_axis',(1.,0.,0.));
#27766=DIRECTION('center_axis',(0.,1.,0.));
#27767=DIRECTION('ref_axis',(1.,0.,0.));
#27768=DIRECTION('',(0.,1.,0.));
#27769=DIRECTION('center_axis',(0.,-1.,0.));
#27770=DIRECTION('ref_axis',(1.,0.,0.));
#27771=DIRECTION('center_axis',(0.,-1.,0.));
#27772=DIRECTION('ref_axis',(1.,0.,0.));
#27773=DIRECTION('center_axis',(0.,-1.,0.));
#27774=DIRECTION('ref_axis',(0.,0.,-1.));
#27775=DIRECTION('center_axis',(-1.,0.,0.));
#27776=DIRECTION('ref_axis',(0.,0.,1.));
#27777=DIRECTION('center_axis',(0.,1.,0.));
#27778=DIRECTION('ref_axis',(0.,0.,1.));
#27779=DIRECTION('center_axis',(-1.,0.,1.22464679914735E-16));
#27780=DIRECTION('ref_axis',(-1.22464679914735E-16,0.,-1.));
#27781=DIRECTION('center_axis',(0.,1.,0.));
#27782=DIRECTION('ref_axis',(1.,0.,0.));
#27783=DIRECTION('center_axis',(0.,1.,0.));
#27784=DIRECTION('ref_axis',(1.,0.,0.));
#27785=DIRECTION('center_axis',(0.,1.,0.));
#27786=DIRECTION('ref_axis',(1.,0.,0.));
#27787=DIRECTION('',(0.,1.,0.));
#27788=DIRECTION('center_axis',(0.,-1.,0.));
#27789=DIRECTION('ref_axis',(1.,0.,0.));
#27790=DIRECTION('center_axis',(0.,-1.,0.));
#27791=DIRECTION('ref_axis',(1.,0.,0.));
#27792=DIRECTION('center_axis',(0.,-1.,0.));
#27793=DIRECTION('ref_axis',(0.,0.,-1.));
#27794=DIRECTION('center_axis',(-1.,0.,-1.22464679914735E-16));
#27795=DIRECTION('ref_axis',(-1.22464679914735E-16,0.,1.));
#27796=DIRECTION('center_axis',(0.,-0.847998304005088,-0.52999894000318));
#27797=DIRECTION('ref_axis',(0.,0.52999894000318,-0.847998304005088));
#27798=DIRECTION('center_axis',(1.,0.,0.));
#27799=DIRECTION('ref_axis',(0.,0.961248746164355,0.275682513042551));
#27800=DIRECTION('',(1.,0.,0.));
#27801=DIRECTION('center_axis',(1.,0.,0.));
#27802=DIRECTION('ref_axis',(0.,-0.961248746164355,-0.275682513042551));
#27803=DIRECTION('',(-1.,0.,0.));
#27804=DIRECTION('center_axis',(0.,0.847998304005088,0.52999894000318));
#27805=DIRECTION('ref_axis',(0.,-0.52999894000318,0.847998304005088));
#97801=CARTESIAN_POINT('',(0.,0.,0.));
#97802=CARTESIAN_POINT('Origin',(12.348,-1.428,45.396));
#97803=CARTESIAN_POINT('',(12.648,0.924,45.396));
#97804=CARTESIAN_POINT('',(12.348,0.924,45.696));
#97805=CARTESIAN_POINT('Origin',(12.348,0.924,45.396));
#97806=CARTESIAN_POINT('',(12.348,0.708,45.696));
#97807=CARTESIAN_POINT('',(12.348,-1.428,45.696));
#97808=CARTESIAN_POINT('',(12.648,0.708,45.396));
#97809=CARTESIAN_POINT('Origin',(12.348,0.708,45.396));
#97810=CARTESIAN_POINT('',(12.648,-1.428,45.396));
#97811=CARTESIAN_POINT('Origin',(0.,0.708,45.396));
#97812=CARTESIAN_POINT('',(-12.348,0.708,45.696));
#97813=CARTESIAN_POINT('',(-12.348,0.408,45.396));
#97814=CARTESIAN_POINT('Origin',(-12.348,0.708,45.396));
#97815=CARTESIAN_POINT('',(12.348,0.408,45.396));
#97816=CARTESIAN_POINT('',(0.,0.408,45.396));
#97817=CARTESIAN_POINT('Origin',(12.348,0.708,45.396));
#97818=CARTESIAN_POINT('',(0.,0.708,45.696));
#97819=CARTESIAN_POINT('Origin',(-12.348,-1.428,45.396));
#97820=CARTESIAN_POINT('',(-12.648,0.708,45.396));
#97821=CARTESIAN_POINT('Origin',(-12.348,0.708,45.396));
#97822=CARTESIAN_POINT('',(-12.348,0.924,45.696));
#97823=CARTESIAN_POINT('',(-12.348,-1.428,45.696));
#97824=CARTESIAN_POINT('',(-12.648,0.924,45.396));
#97825=CARTESIAN_POINT('Origin',(-12.348,0.924,45.396));
#97826=CARTESIAN_POINT('',(-12.648,-1.428,45.396));
#97827=CARTESIAN_POINT('Origin',(0.,0.924,45.396));
#97828=CARTESIAN_POINT('',(12.348,1.224,45.396));
#97829=CARTESIAN_POINT('Origin',(12.348,0.924,45.396));
#97830=CARTESIAN_POINT('',(-12.348,1.224,45.396));
#97831=CARTESIAN_POINT('',(0.,1.224,45.396));
#97832=CARTESIAN_POINT('Origin',(-12.348,0.924,45.396));
#97833=CARTESIAN_POINT('',(0.,0.924,45.696));
#97834=CARTESIAN_POINT('Origin',(-12.348,0.924,45.396));
#97835=CARTESIAN_POINT('Origin',(-12.348,0.924,45.396));
#97836=CARTESIAN_POINT('Origin',(-12.348,0.708,45.396));
#97837=CARTESIAN_POINT('Origin',(-12.348,0.708,45.396));
#97838=CARTESIAN_POINT('Origin',(12.348,0.708,45.396));
#97839=CARTESIAN_POINT('Origin',(12.348,0.708,45.396));
#97840=CARTESIAN_POINT('Origin',(12.348,0.924,45.396));
#97841=CARTESIAN_POINT('Origin',(12.348,0.924,45.396));
#97842=CARTESIAN_POINT('Origin',(-12.348,0.708,43.86));
#97843=CARTESIAN_POINT('',(-12.648,0.708,42.0374493210098));
#97844=CARTESIAN_POINT('',(-12.648,0.708,43.86));
#97845=CARTESIAN_POINT('',(-12.348,0.408,42.0374493210099));
#97846=CARTESIAN_POINT('Origin',(-12.348,0.708,42.0374493210099));
#97847=CARTESIAN_POINT('',(-12.348,0.408,43.86));
#97848=CARTESIAN_POINT('Origin',(-12.648,-4.08,42.024));
#97849=CARTESIAN_POINT('',(-12.648,0.924000000000001,42.0374493210099));
#97850=CARTESIAN_POINT('',(-12.648,0.924,26.4792));
#97851=CARTESIAN_POINT('',(-12.648,0.708,42.03744932101));
#97852=CARTESIAN_POINT('Origin',(-12.348,0.924,26.4792));
#97853=CARTESIAN_POINT('',(-12.348,1.224,42.0374493210099));
#97854=CARTESIAN_POINT('',(-12.348,1.224,26.4792));
#97855=CARTESIAN_POINT('Origin',(-12.348,0.924,42.0374493210099));
#97856=CARTESIAN_POINT('Origin',(0.,1.224,10.9344));
#97857=CARTESIAN_POINT('',(12.348,1.224,42.0374493210129));
#97858=CARTESIAN_POINT('',(12.348,1.224,28.3152));
#97859=CARTESIAN_POINT('',(7.98599766308269,1.224,11.2854385811275));
#97860=CARTESIAN_POINT('Ctrl Pts',(7.98599766308269,1.224,11.2854385811275));
#97861=CARTESIAN_POINT('Ctrl Pts',(8.26166260011058,1.224,12.0417095524849));
#97862=CARTESIAN_POINT('Ctrl Pts',(8.80736065451927,1.224,13.5673576300013));
#97863=CARTESIAN_POINT('Ctrl Pts',(9.7934853134899,1.224,16.6303022412252));
#97864=CARTESIAN_POINT('Ctrl Pts',(10.8098927869894,1.224,19.6660154770441));
#97865=CARTESIAN_POINT('Ctrl Pts',(11.7490851570277,1.224,22.7510694457356));
#97866=CARTESIAN_POINT('Ctrl Pts',(12.3879445445635,1.224,25.0858368018936));
#97867=CARTESIAN_POINT('Ctrl Pts',(12.9162393467085,1.224,27.0283271988516));
#97868=CARTESIAN_POINT('Ctrl Pts',(13.318072367284,1.224,28.3480811193172));
#97869=CARTESIAN_POINT('Ctrl Pts',(13.5413604393248,1.224,29.0034673861264));
#97870=CARTESIAN_POINT('Ctrl Pts',(13.6793149470157,1.224,29.3805129744774));
#97871=CARTESIAN_POINT('Ctrl Pts',(13.8956419055917,1.224,29.9480318039803));
#97872=CARTESIAN_POINT('Ctrl Pts',(14.1903040593961,1.224,30.6134675776983));
#97873=CARTESIAN_POINT('Ctrl Pts',(14.5193620015612,1.224,31.3678458791788));
#97874=CARTESIAN_POINT('Ctrl Pts',(14.711967368694,1.224,31.9396546207724));
#97875=CARTESIAN_POINT('Ctrl Pts',(14.7690013588176,1.224,32.5519725397467));
#97876=CARTESIAN_POINT('Ctrl Pts',(14.5616693526593,1.224,33.1335095406623));
#97877=CARTESIAN_POINT('Ctrl Pts',(14.1770509140562,1.224,33.6045046700376));
#97878=CARTESIAN_POINT('Ctrl Pts',(13.5570600775614,1.224,34.1220294622509));
#97879=CARTESIAN_POINT('Ctrl Pts',(12.6963985226976,1.224,34.6417186073242));
#97880=CARTESIAN_POINT('Ctrl Pts',(11.6986604523811,1.224,35.333270779735));
#97881=CARTESIAN_POINT('Ctrl Pts',(10.9714653585921,1.224,36.3268151158983));
#97882=CARTESIAN_POINT('Ctrl Pts',(10.704924469272,1.224,37.5319055503386));
#97883=CARTESIAN_POINT('Ctrl Pts',(10.8999667707481,1.224,38.7410381732305));
#97884=CARTESIAN_POINT('Ctrl Pts',(11.4452668024532,1.224,39.8274946497674));
#97885=CARTESIAN_POINT('Ctrl Pts',(12.0610698910061,1.224,40.8549578815901));
#97886=CARTESIAN_POINT('Ctrl Pts',(12.3110725606623,1.224,41.6363966051383));
#97887=CARTESIAN_POINT('Ctrl Pts',(12.348,1.224,42.0374493210131));
#97888=CARTESIAN_POINT('',(-7.98599766308436,1.224,11.2854385811275));
#97889=CARTESIAN_POINT('',(0.,1.224,11.2854385811275));
#97890=CARTESIAN_POINT('Ctrl Pts',(-12.348,1.224,42.03744932101));
#97891=CARTESIAN_POINT('Ctrl Pts',(-12.3110725606702,1.224,41.6363966051328));
#97892=CARTESIAN_POINT('Ctrl Pts',(-12.0609852952635,1.224,40.8549204601091));
#97893=CARTESIAN_POINT('Ctrl Pts',(-11.4450821737987,1.224,39.8274092249604));
#97894=CARTESIAN_POINT('Ctrl Pts',(-10.8997688026688,1.224,38.7409075676707));
#97895=CARTESIAN_POINT('Ctrl Pts',(-10.7043533514793,1.224,37.5315890187733));
#97896=CARTESIAN_POINT('Ctrl Pts',(-10.9709851394883,1.224,36.3263525491271));
#97897=CARTESIAN_POINT('Ctrl Pts',(-11.6986135266186,1.224,35.3339416136743));
#97898=CARTESIAN_POINT('Ctrl Pts',(-12.5309171577631,1.224,34.7574741120408));
#97899=CARTESIAN_POINT('Ctrl Pts',(-13.2114636130569,1.224,34.3298336160849));
#97900=CARTESIAN_POINT('Ctrl Pts',(-13.7131082734894,1.224,33.9932968374398));
#97901=CARTESIAN_POINT('Ctrl Pts',(-14.1769757204202,1.224,33.6048339401135));
#97902=CARTESIAN_POINT('Ctrl Pts',(-14.5620228329377,1.224,33.1340383684088));
#97903=CARTESIAN_POINT('Ctrl Pts',(-14.7683961662382,1.224,32.5514380647304));
#97904=CARTESIAN_POINT('Ctrl Pts',(-14.711659402932,1.224,31.939868704061));
#97905=CARTESIAN_POINT('Ctrl Pts',(-14.5189773065471,1.224,31.3678083420515));
#97906=CARTESIAN_POINT('Ctrl Pts',(-14.1888423807734,1.224,30.613847819264));
#97907=CARTESIAN_POINT('Ctrl Pts',(-13.6063457415431,1.224,29.2804450588471));
#97908=CARTESIAN_POINT('Ctrl Pts',(-13.0245909094872,1.224,27.4180026826501));
#97909=CARTESIAN_POINT('Ctrl Pts',(-12.3871316955906,1.224,25.0852094102837));
#97910=CARTESIAN_POINT('Ctrl Pts',(-11.7493811375928,1.224,22.7517028806517));
#97911=CARTESIAN_POINT('Ctrl Pts',(-10.8084555662763,1.224,19.6656582368069));
#97912=CARTESIAN_POINT('Ctrl Pts',(-9.79376320963301,1.224,16.6304717567395));
#97913=CARTESIAN_POINT('Ctrl Pts',(-8.80744652629141,1.224,13.5670274338247));
#97914=CARTESIAN_POINT('Ctrl Pts',(-8.26166260011136,1.224,12.0417095524852));
#97915=CARTESIAN_POINT('Ctrl Pts',(-7.98599766308436,1.224,11.2854385811275));
#97916=CARTESIAN_POINT('',(6.528,1.224,44.032));
#97917=CARTESIAN_POINT('Origin',(6.528,1.224,42.432));
#97918=CARTESIAN_POINT('',(-6.528,1.224,44.032));
#97919=CARTESIAN_POINT('Origin',(-6.528,1.224,42.432));
#97920=CARTESIAN_POINT('Origin',(0.,1.224,45.696));
#97921=CARTESIAN_POINT('Origin',(12.348,0.924,28.3152));
#97922=CARTESIAN_POINT('',(12.648,0.924,42.0374493210128));
#97923=CARTESIAN_POINT('',(12.648,0.924,28.3152));
#97924=CARTESIAN_POINT('Origin',(12.348,0.924,42.0374493210129));
#97925=CARTESIAN_POINT('Origin',(12.3479078516757,0.708,42.0374535543961));
#97926=CARTESIAN_POINT('',(12.646736323466,0.924,42.009942793751));
#97927=CARTESIAN_POINT('Origin',(12.348,0.924,42.037449321013));
#97928=CARTESIAN_POINT('',(12.648,0.708,42.0374493210129));
#97929=CARTESIAN_POINT('',(12.648,0.924,42.037449321013));
#97930=CARTESIAN_POINT('',(12.646736323466,0.708000000000001,42.009942793751));
#97931=CARTESIAN_POINT('Origin',(12.348,0.708,42.037449321013));
#97932=CARTESIAN_POINT('',(12.646736323466,0.708,42.0099427937509));
#97933=CARTESIAN_POINT('Origin',(12.348,0.924,42.037449321013));
#97934=CARTESIAN_POINT('Origin',(12.348,0.924,42.037449321013));
#97935=CARTESIAN_POINT('Origin',(12.348,0.708,45.696));
#97936=CARTESIAN_POINT('',(12.348,0.408,42.0374493210129));
#97937=CARTESIAN_POINT('',(12.348,0.408,45.696));
#97938=CARTESIAN_POINT('Origin',(12.348,0.708,42.0374493210129));
#97939=CARTESIAN_POINT('',(12.648,0.708,45.696));
#97940=CARTESIAN_POINT('Origin',(12.348,0.708,42.037449321013));
#97941=CARTESIAN_POINT('Origin',(12.348,0.708,42.037449321013));
#97942=CARTESIAN_POINT('Ctrl Pts',(7.98599766308269,1.224,11.2854385811275));
#97943=CARTESIAN_POINT('Ctrl Pts',(8.26166260011058,1.224,12.0417095524849));
#97944=CARTESIAN_POINT('Ctrl Pts',(8.80736065451927,1.224,13.5673576300013));
#97945=CARTESIAN_POINT('Ctrl Pts',(9.7934853134899,1.224,16.6303022412252));
#97946=CARTESIAN_POINT('Ctrl Pts',(10.8098927869894,1.224,19.6660154770441));
#97947=CARTESIAN_POINT('Ctrl Pts',(11.7490851570277,1.224,22.7510694457356));
#97948=CARTESIAN_POINT('Ctrl Pts',(12.3879445445635,1.224,25.0858368018936));
#97949=CARTESIAN_POINT('Ctrl Pts',(12.9162393467085,1.224,27.0283271988516));
#97950=CARTESIAN_POINT('Ctrl Pts',(13.318072367284,1.224,28.3480811193172));
#97951=CARTESIAN_POINT('Ctrl Pts',(13.5413604393248,1.224,29.0034673861264));
#97952=CARTESIAN_POINT('Ctrl Pts',(13.6793149470157,1.224,29.3805129744774));
#97953=CARTESIAN_POINT('Ctrl Pts',(13.8956419055917,1.224,29.9480318039803));
#97954=CARTESIAN_POINT('Ctrl Pts',(14.1903040593961,1.224,30.6134675776983));
#97955=CARTESIAN_POINT('Ctrl Pts',(14.5193620015612,1.224,31.3678458791788));
#97956=CARTESIAN_POINT('Ctrl Pts',(14.711967368694,1.224,31.9396546207724));
#97957=CARTESIAN_POINT('Ctrl Pts',(14.7690013588176,1.224,32.5519725397467));
#97958=CARTESIAN_POINT('Ctrl Pts',(14.5616693526593,1.224,33.1335095406623));
#97959=CARTESIAN_POINT('Ctrl Pts',(14.1770509140562,1.224,33.6045046700376));
#97960=CARTESIAN_POINT('Ctrl Pts',(13.5570600775614,1.224,34.1220294622509));
#97961=CARTESIAN_POINT('Ctrl Pts',(12.6963985226976,1.224,34.6417186073242));
#97962=CARTESIAN_POINT('Ctrl Pts',(11.6986604523811,1.224,35.333270779735));
#97963=CARTESIAN_POINT('Ctrl Pts',(10.9714653585921,1.224,36.3268151158983));
#97964=CARTESIAN_POINT('Ctrl Pts',(10.704924469272,1.224,37.5319055503386));
#97965=CARTESIAN_POINT('Ctrl Pts',(10.8999667707481,1.224,38.7410381732305));
#97966=CARTESIAN_POINT('Ctrl Pts',(11.4452668024532,1.224,39.8274946497674));
#97967=CARTESIAN_POINT('Ctrl Pts',(12.0610698910061,1.224,40.8549578815901));
#97968=CARTESIAN_POINT('Ctrl Pts',(12.3110725606623,1.224,41.6363966051383));
#97969=CARTESIAN_POINT('Ctrl Pts',(12.348,1.224,42.0374493210131));
#97970=CARTESIAN_POINT('Ctrl Pts',(8.05978824615337,1.224,11.2585415069228));
#97971=CARTESIAN_POINT('Ctrl Pts',(8.33546863203364,1.224,12.0148310799991));
#97972=CARTESIAN_POINT('Ctrl Pts',(8.88191390907659,1.224,13.5426216579679));
#97973=CARTESIAN_POINT('Ctrl Pts',(9.86823614904903,1.224,16.6062333317922));
#97974=CARTESIAN_POINT('Ctrl Pts',(10.8843947824238,1.224,19.6411006535636));
#97975=CARTESIAN_POINT('Ctrl Pts',(11.8246493128098,1.224,22.7295876128389));
#97976=CARTESIAN_POINT('Ctrl Pts',(12.4637767343052,1.224,25.0654345278681));
#97977=CARTESIAN_POINT('Ctrl Pts',(12.9919022546425,1.224,27.0072148023256));
#97978=CARTESIAN_POINT('Ctrl Pts',(13.39292056091,1.224,28.3242302479708));
#97979=CARTESIAN_POINT('Ctrl Pts',(13.6154785859392,1.224,28.9774817878985));
#97980=CARTESIAN_POINT('Ctrl Pts',(13.7528646368703,1.224,29.3529231195986));
#97981=CARTESIAN_POINT('Ctrl Pts',(13.9683464603798,1.224,29.918401670249));
#97982=CARTESIAN_POINT('Ctrl Pts',(14.2615438634277,1.224,30.5801122589648));
#97983=CARTESIAN_POINT('Ctrl Pts',(14.5921672247916,1.224,31.3385970564082));
#97984=CARTESIAN_POINT('Ctrl Pts',(14.7888026951731,1.224,31.9199846429038));
#97985=CARTESIAN_POINT('Ctrl Pts',(14.8496195982487,1.224,32.5610656869859));
#97986=CARTESIAN_POINT('Ctrl Pts',(14.6302688785353,1.224,33.1755044896258));
#97987=CARTESIAN_POINT('Ctrl Pts',(14.2320817324303,1.224,33.6607769671911));
#97988=CARTESIAN_POINT('Ctrl Pts',(13.6008246044553,1.224,34.1879453054762));
#97989=CARTESIAN_POINT('Ctrl Pts',(12.7358933411632,1.224,34.7091332477064));
#97990=CARTESIAN_POINT('Ctrl Pts',(11.7523239260966,1.224,35.3928958840521));
#97991=CARTESIAN_POINT('Ctrl Pts',(11.0455333850698,1.224,36.3596210864882));
#97992=CARTESIAN_POINT('Ctrl Pts',(10.7852936168046,1.224,37.5340147061541));
#97993=CARTESIAN_POINT('Ctrl Pts',(10.9753230697622,1.224,38.7144559876328));
#97994=CARTESIAN_POINT('Ctrl Pts',(11.5120188762668,1.224,39.7864283699758));
#97995=CARTESIAN_POINT('Ctrl Pts',(12.1314071774355,1.224,40.8188642924511));
#97996=CARTESIAN_POINT('Ctrl Pts',(12.3884534787586,1.224,41.6182742012834));
#97997=CARTESIAN_POINT('Ctrl Pts',(12.4262089865968,1.224,42.0302481290154));
#97998=CARTESIAN_POINT('Ctrl Pts',(8.20673516090132,1.15894437659295,11.2049785466419));
#97999=CARTESIAN_POINT('Ctrl Pts',(8.48246583853968,1.15894437659295,11.9614138362237));
#98000=CARTESIAN_POINT('Ctrl Pts',(9.03031785403706,1.15894437659295,13.493174874988));
#98001=CARTESIAN_POINT('Ctrl Pts',(10.0171159532212,1.15894437659295,16.5583667565347));
#98002=CARTESIAN_POINT('Ctrl Pts',(11.032807640009,1.15894437659295,19.5916239397643));
#98003=CARTESIAN_POINT('Ctrl Pts',(11.9750949600252,1.15894437659295,22.6867145384626));
#98004=CARTESIAN_POINT('Ctrl Pts',(12.6148189226952,1.15894437659295,25.0249062630847));
#98005=CARTESIAN_POINT('Ctrl Pts',(13.1425604647687,1.15894437659295,26.9651479861995));
#98006=CARTESIAN_POINT('Ctrl Pts',(13.5419982523509,1.15894437659294,28.276870675056));
#98007=CARTESIAN_POINT('Ctrl Pts',(13.7630823643497,1.15894437659294,28.9257801857052));
#98008=CARTESIAN_POINT('Ctrl Pts',(13.8993694172056,1.15894437659294,29.2982183234201));
#98009=CARTESIAN_POINT('Ctrl Pts',(14.1130820755258,1.15894437659295,29.8590949099225));
#98010=CARTESIAN_POINT('Ctrl Pts',(14.4033529215945,1.15894437659295,30.5138988935207));
#98011=CARTESIAN_POINT('Ctrl Pts',(14.7371296392622,1.15894437659295,31.27998110634));
#98012=CARTESIAN_POINT('Ctrl Pts',(14.941677315901,1.15894437659295,31.8806320069506));
#98013=CARTESIAN_POINT('Ctrl Pts',(15.0102531276634,1.15894437659295,32.5790650964589));
#98014=CARTESIAN_POINT('Ctrl Pts',(14.7668033293489,1.15894437659295,33.2588822083198));
#98015=CARTESIAN_POINT('Ctrl Pts',(14.3419892667217,1.15894437659295,33.772786749341));
#98016=CARTESIAN_POINT('Ctrl Pts',(13.687845201664,1.15894437659295,34.3192421394686));
#98017=CARTESIAN_POINT('Ctrl Pts',(12.814864656712,1.15894437659295,34.8436494734496));
#98018=CARTESIAN_POINT('Ctrl Pts',(11.8591318733617,1.15894437659295,35.5117504800206));
#98019=CARTESIAN_POINT('Ctrl Pts',(11.192774610864,1.15894437659295,36.4248976115355));
#98020=CARTESIAN_POINT('Ctrl Pts',(10.945224692698,1.15894437659295,37.5383568976139));
#98021=CARTESIAN_POINT('Ctrl Pts',(11.1252475782242,1.15894437659295,38.6613956307185));
#98022=CARTESIAN_POINT('Ctrl Pts',(11.6448524105777,1.15894437659295,39.7049780164935));
#98023=CARTESIAN_POINT('Ctrl Pts',(12.2714401993632,1.15894437659295,40.7466056673881));
#98024=CARTESIAN_POINT('Ctrl Pts',(12.5422016913503,1.15894437659295,41.582867190141));
#98025=CARTESIAN_POINT('Ctrl Pts',(12.5819547309413,1.15894437659295,42.0159076413469));
#98026=CARTESIAN_POINT('Ctrl Pts',(8.26785692826664,1.00253981633974,11.1826993255823));
#98027=CARTESIAN_POINT('Ctrl Pts',(8.543613066273,1.00253981633974,11.9392205016025));
#98028=CARTESIAN_POINT('Ctrl Pts',(9.09203130090063,1.00253981633974,13.4725641556529));
#98029=CARTESIAN_POINT('Ctrl Pts',(10.0790464956501,1.00253981633974,16.5384718863773));
#98030=CARTESIAN_POINT('Ctrl Pts',(11.0945506094751,1.00253981633974,19.5710766504504));
#98031=CARTESIAN_POINT('Ctrl Pts',(12.0376642913239,1.00253981633974,22.6688598415768));
#98032=CARTESIAN_POINT('Ctrl Pts',(12.677650983484,1.00253981633974,25.00807222563));
#98033=CARTESIAN_POINT('Ctrl Pts',(13.2052219103856,1.00253981633974,26.9476450599348));
#98034=CARTESIAN_POINT('Ctrl Pts',(13.6040120371276,1.00253981633974,28.2572036225122));
#98035=CARTESIAN_POINT('Ctrl Pts',(13.8244784093479,1.00253981633974,28.9042859415608));
#98036=CARTESIAN_POINT('Ctrl Pts',(13.9603160223219,1.00253981633974,29.2755194655201));
#98037=CARTESIAN_POINT('Ctrl Pts',(14.1732727660916,1.00253981633974,29.8343565362973));
#98038=CARTESIAN_POINT('Ctrl Pts',(14.4623240833064,1.00253981633974,30.4864067831395));
#98039=CARTESIAN_POINT('Ctrl Pts',(14.7974207893837,1.00253981633974,31.2555141309736));
#98040=CARTESIAN_POINT('Ctrl Pts',(15.0052331383414,1.00253981633974,31.8642212193198));
#98041=CARTESIAN_POINT('Ctrl Pts',(15.0770886981136,1.00253981633974,32.586526563643));
#98042=CARTESIAN_POINT('Ctrl Pts',(14.8235766521624,1.00253981633974,33.2935042835916));
#98043=CARTESIAN_POINT('Ctrl Pts',(14.3877788802376,1.00253981633974,33.8193647133348));
#98044=CARTESIAN_POINT('Ctrl Pts',(13.7240101751605,1.00253981633974,34.3738617173899));
#98045=CARTESIAN_POINT('Ctrl Pts',(12.8477870409378,1.00253981633974,34.8996627244856));
#98046=CARTESIAN_POINT('Ctrl Pts',(11.9035446247143,1.00253981633974,35.5612145865672));
#98047=CARTESIAN_POINT('Ctrl Pts',(11.2539587421444,1.00253981633974,36.4520365963864));
#98048=CARTESIAN_POINT('Ctrl Pts',(11.0117200719654,1.00253981633974,37.5401960385209));
#98049=CARTESIAN_POINT('Ctrl Pts',(11.1875752081005,1.00253981633975,38.6392965146994));
#98050=CARTESIAN_POINT('Ctrl Pts',(11.7000812655187,1.00253981633974,39.6711757625401));
#98051=CARTESIAN_POINT('Ctrl Pts',(12.3296775691092,1.00253981633975,40.7164613105102));
#98052=CARTESIAN_POINT('Ctrl Pts',(12.6060713603057,1.00253981633974,41.5682984715638));
#98053=CARTESIAN_POINT('Ctrl Pts',(12.646736323466,1.00253981633974,42.0099427937509));
#98054=CARTESIAN_POINT('Ctrl Pts',(8.26785692826664,0.923999999999997,11.1826993255823));
#98055=CARTESIAN_POINT('Ctrl Pts',(8.543613066273,0.923999999999997,11.9392205016025));
#98056=CARTESIAN_POINT('Ctrl Pts',(9.09203130090063,0.924,13.4725641556529));
#98057=CARTESIAN_POINT('Ctrl Pts',(10.0790464956501,0.923999999999999,16.5384718863773));
#98058=CARTESIAN_POINT('Ctrl Pts',(11.0945506094751,0.924,19.5710766504504));
#98059=CARTESIAN_POINT('Ctrl Pts',(12.0376642913239,0.924,22.6688598415768));
#98060=CARTESIAN_POINT('Ctrl Pts',(12.677650983484,0.924,25.00807222563));
#98061=CARTESIAN_POINT('Ctrl Pts',(13.2052219103856,0.923999999999999,26.9476450599348));
#98062=CARTESIAN_POINT('Ctrl Pts',(13.6040120371276,0.923999999999998,28.2572036225122));
#98063=CARTESIAN_POINT('Ctrl Pts',(13.8244784093479,0.923999999999997,28.9042859415608));
#98064=CARTESIAN_POINT('Ctrl Pts',(13.9603160223219,0.923999999999998,29.2755194655201));
#98065=CARTESIAN_POINT('Ctrl Pts',(14.1732727660916,0.923999999999998,29.8343565362973));
#98066=CARTESIAN_POINT('Ctrl Pts',(14.4623240833064,0.923999999999999,30.4864067831395));
#98067=CARTESIAN_POINT('Ctrl Pts',(14.7974207893837,0.923999999999999,31.2555141309736));
#98068=CARTESIAN_POINT('Ctrl Pts',(15.0052331383414,0.923999999999999,31.8642212193198));
#98069=CARTESIAN_POINT('Ctrl Pts',(15.0770886981136,0.923999999999999,32.586526563643));
#98070=CARTESIAN_POINT('Ctrl Pts',(14.8235766521624,0.924,33.2935042835916));
#98071=CARTESIAN_POINT('Ctrl Pts',(14.3877788802376,0.924,33.8193647133348));
#98072=CARTESIAN_POINT('Ctrl Pts',(13.7240101751605,0.924,34.3738617173899));
#98073=CARTESIAN_POINT('Ctrl Pts',(12.8477870409378,0.924,34.8996627244856));
#98074=CARTESIAN_POINT('Ctrl Pts',(11.9035446247143,0.924,35.5612145865672));
#98075=CARTESIAN_POINT('Ctrl Pts',(11.2539587421444,0.924,36.4520365963864));
#98076=CARTESIAN_POINT('Ctrl Pts',(11.0117200719654,0.924,37.5401960385209));
#98077=CARTESIAN_POINT('Ctrl Pts',(11.1875752081005,0.924,38.6392965146994));
#98078=CARTESIAN_POINT('Ctrl Pts',(11.7000812655187,0.924,39.6711757625401));
#98079=CARTESIAN_POINT('Ctrl Pts',(12.3296775691092,0.924,40.7164613105102));
#98080=CARTESIAN_POINT('Ctrl Pts',(12.6060713603057,0.924,41.5682984715638));
#98081=CARTESIAN_POINT('Ctrl Pts',(12.646736323466,0.924,42.0099427937509));
#98082=CARTESIAN_POINT('',(8.26785692826664,0.924,11.1826993255823));
#98083=CARTESIAN_POINT('Ctrl Pts',(12.646736323466,0.924,42.0099427937509));
#98084=CARTESIAN_POINT('Ctrl Pts',(12.6060713603057,0.924,41.5682984715638));
#98085=CARTESIAN_POINT('Ctrl Pts',(12.3296775691092,0.924,40.7164613105102));
#98086=CARTESIAN_POINT('Ctrl Pts',(11.7000812655187,0.924,39.6711757625401));
#98087=CARTESIAN_POINT('Ctrl Pts',(11.1875752081005,0.924,38.6392965146994));
#98088=CARTESIAN_POINT('Ctrl Pts',(11.0117200719654,0.924,37.5401960385209));
#98089=CARTESIAN_POINT('Ctrl Pts',(11.2539587421444,0.924,36.4520365963864));
#98090=CARTESIAN_POINT('Ctrl Pts',(11.9035446247143,0.924,35.5612145865672));
#98091=CARTESIAN_POINT('Ctrl Pts',(12.8477870409378,0.924,34.8996627244856));
#98092=CARTESIAN_POINT('Ctrl Pts',(13.7240101751605,0.924,34.3738617173899));
#98093=CARTESIAN_POINT('Ctrl Pts',(14.3877788802376,0.924,33.8193647133348));
#98094=CARTESIAN_POINT('Ctrl Pts',(14.8235766521624,0.924,33.2935042835916));
#98095=CARTESIAN_POINT('Ctrl Pts',(15.0770886981136,0.923999999999999,32.586526563643));
#98096=CARTESIAN_POINT('Ctrl Pts',(15.0052331383414,0.923999999999999,31.8642212193198));
#98097=CARTESIAN_POINT('Ctrl Pts',(14.7974207893837,0.923999999999999,31.2555141309736));
#98098=CARTESIAN_POINT('Ctrl Pts',(14.4623240833064,0.923999999999999,30.4864067831395));
#98099=CARTESIAN_POINT('Ctrl Pts',(14.1732727660916,0.923999999999998,29.8343565362973));
#98100=CARTESIAN_POINT('Ctrl Pts',(13.9603160223219,0.923999999999998,29.2755194655201));
#98101=CARTESIAN_POINT('Ctrl Pts',(13.8244784093479,0.923999999999997,28.9042859415608));
#98102=CARTESIAN_POINT('Ctrl Pts',(13.6040120371276,0.923999999999998,28.2572036225122));
#98103=CARTESIAN_POINT('Ctrl Pts',(13.2052219103856,0.923999999999999,26.9476450599348));
#98104=CARTESIAN_POINT('Ctrl Pts',(12.677650983484,0.924,25.00807222563));
#98105=CARTESIAN_POINT('Ctrl Pts',(12.0376642913239,0.924,22.6688598415768));
#98106=CARTESIAN_POINT('Ctrl Pts',(11.0945506094751,0.924,19.5710766504504));
#98107=CARTESIAN_POINT('Ctrl Pts',(10.0790464956501,0.923999999999999,16.5384718863773));
#98108=CARTESIAN_POINT('Ctrl Pts',(9.09203130090063,0.924,13.4725641556529));
#98109=CARTESIAN_POINT('Ctrl Pts',(8.543613066273,0.923999999999997,11.9392205016025));
#98110=CARTESIAN_POINT('Ctrl Pts',(8.26785692826664,0.923999999999997,11.1826993255823));
#98111=CARTESIAN_POINT('Origin',(7.98599766308269,0.924,11.2854385811275));
#98112=CARTESIAN_POINT('Ctrl Pts',(12.648,-4.08,42.024));
#98113=CARTESIAN_POINT('Ctrl Pts',(12.648,10.608,42.024));
#98114=CARTESIAN_POINT('Ctrl Pts',(12.641053196814,-4.08,41.9448017311235));
#98115=CARTESIAN_POINT('Ctrl Pts',(12.641053196814,10.608,41.9448017311235));
#98116=CARTESIAN_POINT('Ctrl Pts',(12.6222832973035,-4.08,41.7862967053182));
#98117=CARTESIAN_POINT('Ctrl Pts',(12.6222832973035,10.608,41.7862967053182));
#98118=CARTESIAN_POINT('Ctrl Pts',(12.5795001090523,-4.08,41.5482135599818));
#98119=CARTESIAN_POINT('Ctrl Pts',(12.5795001090523,10.608,41.5482135599818));
#98120=CARTESIAN_POINT('Ctrl Pts',(12.4931832123772,-4.08,41.2301191386837));
#98121=CARTESIAN_POINT('Ctrl Pts',(12.4931832123772,10.608,41.2301191386837));
#98122=CARTESIAN_POINT('Ctrl Pts',(12.3384198670333,-4.08,40.8311101407486));
#98123=CARTESIAN_POINT('Ctrl Pts',(12.3384198670333,10.608,40.8311101407486));
#98124=CARTESIAN_POINT('Ctrl Pts',(12.1425787135413,-4.08,40.4298136303283));
#98125=CARTESIAN_POINT('Ctrl Pts',(12.1425787135413,10.608,40.4298136303283));
#98126=CARTESIAN_POINT('Ctrl Pts',(11.9174888407591,-4.08,40.024395675874));
#98127=CARTESIAN_POINT('Ctrl Pts',(11.9174888407591,10.608,40.024395675874));
#98128=CARTESIAN_POINT('Ctrl Pts',(11.6825137471499,-4.08,39.6119151152301));
#98129=CARTESIAN_POINT('Ctrl Pts',(11.6825137471499,10.608,39.6119151152301));
#98130=CARTESIAN_POINT('Ctrl Pts',(11.4604343652151,-4.08,39.1895865074125));
#98131=CARTESIAN_POINT('Ctrl Pts',(11.4604343652151,10.608,39.1895865074125));
#98132=CARTESIAN_POINT('Ctrl Pts',(11.2737132025486,-4.08,38.7559673641863));
#98133=CARTESIAN_POINT('Ctrl Pts',(11.2737132025486,10.608,38.7559673641863));
#98134=CARTESIAN_POINT('Ctrl Pts',(11.1408514716204,-4.08,38.3120740300016));
#98135=CARTESIAN_POINT('Ctrl Pts',(11.1408514716204,10.608,38.3120740300016));
#98136=CARTESIAN_POINT('Ctrl Pts',(11.0720880317828,-4.08,37.8627943234146));
#98137=CARTESIAN_POINT('Ctrl Pts',(11.0720880317828,10.608,37.8627943234146));
#98138=CARTESIAN_POINT('Ctrl Pts',(11.0709679278862,-4.08,37.4158119459997));
#98139=CARTESIAN_POINT('Ctrl Pts',(11.0709679278862,10.608,37.4158119459997));
#98140=CARTESIAN_POINT('Ctrl Pts',(11.1371764695442,-4.08,36.9800311993457));
#98141=CARTESIAN_POINT('Ctrl Pts',(11.1371764695442,10.608,36.9800311993457));
#98142=CARTESIAN_POINT('Ctrl Pts',(11.2687034908357,-4.08,36.5642101034699));
#98143=CARTESIAN_POINT('Ctrl Pts',(11.2687034908357,10.608,36.5642101034699));
#98144=CARTESIAN_POINT('Ctrl Pts',(11.464839430664,-4.08,36.1754277041587));
#98145=CARTESIAN_POINT('Ctrl Pts',(11.464839430664,10.608,36.1754277041587));
#98146=CARTESIAN_POINT('Ctrl Pts',(11.7250208885943,-4.08,35.8180786547663));
#98147=CARTESIAN_POINT('Ctrl Pts',(11.7250208885943,10.608,35.8180786547663));
#98148=CARTESIAN_POINT('Ctrl Pts',(12.0463519007611,-4.08,35.4928858294797));
#98149=CARTESIAN_POINT('Ctrl Pts',(12.0463519007611,10.608,35.4928858294797));
#98150=CARTESIAN_POINT('Ctrl Pts',(12.4217894296778,-4.08,35.1961083216786));
#98151=CARTESIAN_POINT('Ctrl Pts',(12.4217894296778,10.608,35.1961083216786));
#98152=CARTESIAN_POINT('Ctrl Pts',(12.8374851087503,-4.08,34.9181535900632));
#98153=CARTESIAN_POINT('Ctrl Pts',(12.8374851087503,10.608,34.9181535900632));
#98154=CARTESIAN_POINT('Ctrl Pts',(13.2738213034495,-4.08,34.6454993802755));
#98155=CARTESIAN_POINT('Ctrl Pts',(13.2738213034495,10.608,34.6454993802755));
#98156=CARTESIAN_POINT('Ctrl Pts',(13.7077402642196,-4.08,34.3639065568125));
#98157=CARTESIAN_POINT('Ctrl Pts',(13.7077402642196,10.608,34.3639065568125));
#98158=CARTESIAN_POINT('Ctrl Pts',(14.1146548169614,-4.08,34.0610864824012));
#98159=CARTESIAN_POINT('Ctrl Pts',(14.1146548169614,10.608,34.0610864824012));
#98160=CARTESIAN_POINT('Ctrl Pts',(14.4705118919346,-4.08,33.7298729261479));
#98161=CARTESIAN_POINT('Ctrl Pts',(14.4705118919346,10.608,33.7298729261479));
#98162=CARTESIAN_POINT('Ctrl Pts',(14.7538514224949,-4.08,33.3703634670861));
#98163=CARTESIAN_POINT('Ctrl Pts',(14.7538514224949,10.608,33.3703634670861));
#98164=CARTESIAN_POINT('Ctrl Pts',(14.9484729279409,-4.08,32.9871564326143));
#98165=CARTESIAN_POINT('Ctrl Pts',(14.9484729279409,10.608,32.9871564326143));
#98166=CARTESIAN_POINT('Ctrl Pts',(15.0458732472955,-4.08,32.5872458409767));
#98167=CARTESIAN_POINT('Ctrl Pts',(15.0458732472955,10.608,32.5872458409767));
#98168=CARTESIAN_POINT('Ctrl Pts',(15.0480973104188,-4.08,32.1776017680613));
#98169=CARTESIAN_POINT('Ctrl Pts',(15.0480973104188,10.608,32.1776017680613));
#98170=CARTESIAN_POINT('Ctrl Pts',(14.9695221769895,-4.08,31.7630680429362));
#98171=CARTESIAN_POINT('Ctrl Pts',(14.9695221769895,10.608,31.7630680429362));
#98172=CARTESIAN_POINT('Ctrl Pts',(14.8310295566835,-4.08,31.345457108689));
#98173=CARTESIAN_POINT('Ctrl Pts',(14.8310295566835,10.608,31.345457108689));
#98174=CARTESIAN_POINT('Ctrl Pts',(14.6552019413825,-4.08,30.9226538837489));
#98175=CARTESIAN_POINT('Ctrl Pts',(14.6552019413825,10.608,30.9226538837489));
#98176=CARTESIAN_POINT('Ctrl Pts',(14.4606799971796,-4.08,30.4874491673258));
#98177=CARTESIAN_POINT('Ctrl Pts',(14.4606799971796,10.608,30.4874491673258));
#98178=CARTESIAN_POINT('Ctrl Pts',(14.2582197141431,-4.08,30.0272537125157));
#98179=CARTESIAN_POINT('Ctrl Pts',(14.2582197141431,10.608,30.0272537125157));
#98180=CARTESIAN_POINT('Ctrl Pts',(14.0530623083977,-4.08,29.527374209947));
#98181=CARTESIAN_POINT('Ctrl Pts',(14.0530623083977,10.608,29.527374209947));
#98182=CARTESIAN_POINT('Ctrl Pts',(13.846419362806,-4.08,28.9738645264781));
#98183=CARTESIAN_POINT('Ctrl Pts',(13.846419362806,10.608,28.9738645264781));
#98184=CARTESIAN_POINT('Ctrl Pts',(13.6372170146976,-4.08,28.3563238803391));
#98185=CARTESIAN_POINT('Ctrl Pts',(13.6372170146976,10.608,28.3563238803391));
#98186=CARTESIAN_POINT('Ctrl Pts',(13.4239120315548,-4.08,27.6712450999957));
#98187=CARTESIAN_POINT('Ctrl Pts',(13.4239120315548,10.608,27.6712450999957));
#98188=CARTESIAN_POINT('Ctrl Pts',(13.2056470980329,-4.08,26.9233802340016));
#98189=CARTESIAN_POINT('Ctrl Pts',(13.2056470980329,10.608,26.9233802340016));
#98190=CARTESIAN_POINT('Ctrl Pts',(12.9819542120748,-4.08,26.1231223827782));
#98191=CARTESIAN_POINT('Ctrl Pts',(12.9819542120748,10.608,26.1231223827782));
#98192=CARTESIAN_POINT('Ctrl Pts',(12.7527764582699,-4.08,25.2847489984795));
#98193=CARTESIAN_POINT('Ctrl Pts',(12.7527764582699,10.608,25.2847489984795));
#98194=CARTESIAN_POINT('Ctrl Pts',(12.5183627807979,-4.08,24.4243412707547));
#98195=CARTESIAN_POINT('Ctrl Pts',(12.5183627807979,10.608,24.4243412707547));
#98196=CARTESIAN_POINT('Ctrl Pts',(12.2792174635073,-4.08,23.5578155700232));
#98197=CARTESIAN_POINT('Ctrl Pts',(12.2792174635073,10.608,23.5578155700232));
#98198=CARTESIAN_POINT('Ctrl Pts',(12.0360270133741,-4.08,22.6989792594677));
#98199=CARTESIAN_POINT('Ctrl Pts',(12.0360270133741,10.608,22.6989792594677));
#98200=CARTESIAN_POINT('Ctrl Pts',(11.7895961018279,-4.08,21.8574023995585));
#98201=CARTESIAN_POINT('Ctrl Pts',(11.7895961018279,10.608,21.8574023995585));
#98202=CARTESIAN_POINT('Ctrl Pts',(11.5407830377121,-4.08,21.0368752434048));
#98203=CARTESIAN_POINT('Ctrl Pts',(11.5407830377121,10.608,21.0368752434048));
#98204=CARTESIAN_POINT('Ctrl Pts',(11.2904565074992,-4.08,20.2370106667995));
#98205=CARTESIAN_POINT('Ctrl Pts',(11.2904565074992,10.608,20.2370106667995));
#98206=CARTESIAN_POINT('Ctrl Pts',(11.0394491705041,-4.08,19.4544416356463));
#98207=CARTESIAN_POINT('Ctrl Pts',(11.0394491705041,10.608,19.4544416356463));
#98208=CARTESIAN_POINT('Ctrl Pts',(10.7885123454296,-4.08,18.6841717409459));
#98209=CARTESIAN_POINT('Ctrl Pts',(10.7885123454296,10.608,18.6841717409459));
#98210=CARTESIAN_POINT('Ctrl Pts',(10.53827045241,-4.08,17.9208535267659));
#98211=CARTESIAN_POINT('Ctrl Pts',(10.53827045241,10.608,17.9208535267659));
#98212=CARTESIAN_POINT('Ctrl Pts',(10.2891746222216,-4.08,17.1601046394454));
#98213=CARTESIAN_POINT('Ctrl Pts',(10.2891746222216,10.608,17.1601046394454));
#98214=CARTESIAN_POINT('Ctrl Pts',(10.0414581777664,-4.08,16.3997893456003));
#98215=CARTESIAN_POINT('Ctrl Pts',(10.0414581777664,10.608,16.3997893456003));
#98216=CARTESIAN_POINT('Ctrl Pts',(9.79508602811751,-4.08,15.6413708166744));
#98217=CARTESIAN_POINT('Ctrl Pts',(9.79508602811751,10.608,15.6413708166744));
#98218=CARTESIAN_POINT('Ctrl Pts',(9.5499270515922,-4.08,14.8889496617949));
#98219=CARTESIAN_POINT('Ctrl Pts',(9.5499270515922,10.608,14.8889496617949));
#98220=CARTESIAN_POINT('Ctrl Pts',(9.30593478897464,-4.08,14.1482310979355));
#98221=CARTESIAN_POINT('Ctrl Pts',(9.30593478897464,10.608,14.1482310979355));
#98222=CARTESIAN_POINT('Ctrl Pts',(9.06332174046596,-4.08,13.4255332425459));
#98223=CARTESIAN_POINT('Ctrl Pts',(9.06332174046596,10.608,13.4255332425459));
#98224=CARTESIAN_POINT('Ctrl Pts',(8.8227443525195,-4.08,12.7267521352114));
#98225=CARTESIAN_POINT('Ctrl Pts',(8.8227443525195,10.608,12.7267521352114));
#98226=CARTESIAN_POINT('Ctrl Pts',(8.58546625544561,-4.08,12.0564083534334));
#98227=CARTESIAN_POINT('Ctrl Pts',(8.58546625544561,10.608,12.0564083534334));
#98228=CARTESIAN_POINT('Ctrl Pts',(8.35357461247668,-4.08,11.4165038934492));
#98229=CARTESIAN_POINT('Ctrl Pts',(8.35357461247668,10.608,11.4165038934492));
#98230=CARTESIAN_POINT('Ctrl Pts',(8.13003837378074,-4.08,10.8059423150097));
#98231=CARTESIAN_POINT('Ctrl Pts',(8.13003837378074,10.608,10.8059423150097));
#98232=CARTESIAN_POINT('Ctrl Pts',(7.91830414509172,-4.08,10.2215845279223));
#98233=CARTESIAN_POINT('Ctrl Pts',(7.91830414509172,10.608,10.2215845279223));
#98234=CARTESIAN_POINT('Ctrl Pts',(7.72198141303743,-4.08,9.65899621297674));
#98235=CARTESIAN_POINT('Ctrl Pts',(7.72198141303743,10.608,9.65899621297674));
#98236=CARTESIAN_POINT('Ctrl Pts',(7.54448066029805,-4.08,9.1133393417742));
#98237=CARTESIAN_POINT('Ctrl Pts',(7.54448066029805,10.608,9.1133393417742));
#98238=CARTESIAN_POINT('Ctrl Pts',(7.38869925602481,-4.08,8.58014320427039));
#98239=CARTESIAN_POINT('Ctrl Pts',(7.38869925602481,10.608,8.58014320427039));
#98240=CARTESIAN_POINT('Ctrl Pts',(7.25661399291181,-4.08,8.05627564240542));
#98241=CARTESIAN_POINT('Ctrl Pts',(7.25661399291181,10.608,8.05627564240542));
#98242=CARTESIAN_POINT('Ctrl Pts',(7.14936655485922,-4.08,7.53989292370001));
#98243=CARTESIAN_POINT('Ctrl Pts',(7.14936655485922,10.608,7.53989292370001));
#98244=CARTESIAN_POINT('Ctrl Pts',(7.08388326066375,-4.08,7.13202122230479));
#98245=CARTESIAN_POINT('Ctrl Pts',(7.08388326066375,10.608,7.13202122230479));
#98246=CARTESIAN_POINT('Ctrl Pts',(7.04627094532923,-4.08,6.82892101237943));
#98247=CARTESIAN_POINT('Ctrl Pts',(7.04627094532923,10.608,6.82892101237943));
#98248=CARTESIAN_POINT('Ctrl Pts',(7.02630542760751,-4.08,6.62809945147867));
#98249=CARTESIAN_POINT('Ctrl Pts',(7.02630542760751,10.608,6.62809945147867));
#98250=CARTESIAN_POINT('Ctrl Pts',(7.0176,-4.08,6.528));
#98251=CARTESIAN_POINT('Ctrl Pts',(7.0176,10.608,6.528));
#98252=CARTESIAN_POINT('',(8.14898645568258,0.708,10.8564616996591));
#98253=CARTESIAN_POINT('Ctrl Pts',(8.14898645568258,0.708,10.8564616996591));
#98254=CARTESIAN_POINT('Ctrl Pts',(8.42682850339849,0.708,11.6200722130095));
#98255=CARTESIAN_POINT('Ctrl Pts',(9.00124539599189,0.708,13.1989442398348));
#98256=CARTESIAN_POINT('Ctrl Pts',(10.0164790416783,0.708,16.3416950229929));
#98257=CARTESIAN_POINT('Ctrl Pts',(11.0099910748761,0.708,19.3240277115474));
#98258=CARTESIAN_POINT('Ctrl Pts',(11.9597260958242,0.708,22.3963108112752));
#98259=CARTESIAN_POINT('Ctrl Pts',(12.5087951337059,0.708,24.3892412418576));
#98260=CARTESIAN_POINT('Ctrl Pts',(12.9454833732632,0.708,25.9917673847204));
#98261=CARTESIAN_POINT('Ctrl Pts',(13.3905704701645,0.708,27.5812925495815));
#98262=CARTESIAN_POINT('Ctrl Pts',(13.8494654471821,0.708,29.0499451471956));
#98263=CARTESIAN_POINT('Ctrl Pts',(14.4628824756264,0.708,30.5144902537932));
#98264=CARTESIAN_POINT('Ctrl Pts',(14.8791134736059,0.708,31.4019992941433));
#98265=CARTESIAN_POINT('Ctrl Pts',(15.0241066822088,0.708,32.072069761124));
#98266=CARTESIAN_POINT('Ctrl Pts',(15.0561190850721,0.708,32.5519007446637));
#98267=CARTESIAN_POINT('Ctrl Pts',(14.8974552701336,0.708,33.1680022242259));
#98268=CARTESIAN_POINT('Ctrl Pts',(14.4744331847702,0.708,33.7318712545294));
#98269=CARTESIAN_POINT('Ctrl Pts',(13.8144693967793,0.708,34.3132874952525));
#98270=CARTESIAN_POINT('Ctrl Pts',(12.9271273497437,0.708,34.8526242972181));
#98271=CARTESIAN_POINT('Ctrl Pts',(11.9610261122155,0.708,35.5093720750203));
#98272=CARTESIAN_POINT('Ctrl Pts',(11.2776408422597,0.708,36.3939284497855));
#98273=CARTESIAN_POINT('Ctrl Pts',(11.0124943973279,0.708,37.4880654661885));
#98274=CARTESIAN_POINT('Ctrl Pts',(11.1732013451346,0.708000000000001,38.6029112675029));
#98275=CARTESIAN_POINT('Ctrl Pts',(11.6860758153009,0.708000000000001,39.6451967054032));
#98276=CARTESIAN_POINT('Ctrl Pts',(12.2174359085071,0.708000000000002,40.5301422030716));
#98277=CARTESIAN_POINT('Ctrl Pts',(12.5379284974733,0.708000000000002,41.3444114032542));
#98278=CARTESIAN_POINT('Ctrl Pts',(12.626182924755,0.708000000000003,41.7867213486322));
#98279=CARTESIAN_POINT('Ctrl Pts',(12.646736323466,0.708000000000003,42.0099427937509));
#98280=CARTESIAN_POINT('',(7.97249537063514,0.848449567099299,10.3682028984962));
#98281=CARTESIAN_POINT('Ctrl Pts',(7.97249537063515,0.8484495670993,10.3682028984962));
#98282=CARTESIAN_POINT('Ctrl Pts',(7.99114484243814,0.815737457406984,10.4202957778083));
#98283=CARTESIAN_POINT('Ctrl Pts',(8.01093169220768,0.788564609464305,10.4753461577291));
#98284=CARTESIAN_POINT('Ctrl Pts',(8.03148980819837,0.767115793117118,10.5323403272196));
#98285=CARTESIAN_POINT('Ctrl Pts',(8.05105340780021,0.746704581547924,10.586577355168));
#98286=CARTESIAN_POINT('Ctrl Pts',(8.07131517713305,0.731476987267821,10.642575146733));
#98287=CARTESIAN_POINT('Ctrl Pts',(8.09193208585319,0.721592241216325,10.6994226011466));
#98288=CARTESIAN_POINT('Ctrl Pts',(8.11074776377252,0.712571092578381,10.7513034823833));
#98289=CARTESIAN_POINT('Ctrl Pts',(8.12985877118522,0.708,10.8038918993056));
#98290=CARTESIAN_POINT('Ctrl Pts',(8.14898645568256,0.708,10.8564616996591));
#98291=CARTESIAN_POINT('',(7.19430053092001,2.51634941530375,7.74120895321939));
#98292=CARTESIAN_POINT('Ctrl Pts',(7.19430053092001,2.51634941530375,7.74120895321939));
#98293=CARTESIAN_POINT('Ctrl Pts',(7.37274783895485,1.95099709579208,8.62351966308874));
#98294=CARTESIAN_POINT('Ctrl Pts',(7.65957903289365,1.3973205309983,9.49414527429423));
#98295=CARTESIAN_POINT('Ctrl Pts',(7.97249537063514,0.848449567099299,10.3682028984962));
#98296=CARTESIAN_POINT('',(7.06369006012584,2.748,6.95461383265853));
#98297=CARTESIAN_POINT('Ctrl Pts',(7.06369006012584,2.748,6.95461383265853));
#98298=CARTESIAN_POINT('Ctrl Pts',(7.07278956030561,2.748,7.0252168756328));
#98299=CARTESIAN_POINT('Ctrl Pts',(7.08259944156938,2.74270356870423,7.09569043605442));
#98300=CARTESIAN_POINT('Ctrl Pts',(7.09299220344838,2.73232722308212,7.16540040552519));
#98301=CARTESIAN_POINT('Ctrl Pts',(7.1035593690914,2.72177674918165,7.23628019695548));
#98302=CARTESIAN_POINT('Ctrl Pts',(7.11472903256084,2.70597443554641,7.30637055164591));
#98303=CARTESIAN_POINT('Ctrl Pts',(7.12631318750442,2.68514788338026,7.37499313226435));
#98304=CARTESIAN_POINT('Ctrl Pts',(7.13851349793525,2.66321357717764,7.44726571409596));
#98305=CARTESIAN_POINT('Ctrl Pts',(7.15117348734242,2.63570634471393,7.51791031719418));
#98306=CARTESIAN_POINT('Ctrl Pts',(7.16401500155562,2.60289207116545,7.58612079978413));
#98307=CARTESIAN_POINT('Ctrl Pts',(7.17405198241766,2.57724429862555,7.63943439637247));
#98308=CARTESIAN_POINT('Ctrl Pts',(7.18419849695384,2.54835442786152,7.69126069197653));
#98309=CARTESIAN_POINT('Ctrl Pts',(7.19430053092,2.51634941530376,7.74120895321938));
#98310=CARTESIAN_POINT('',(7.0176,2.748,6.528));
#98311=CARTESIAN_POINT('Origin',(17.3375887917909,2.748,5.6288564499836));
#98312=CARTESIAN_POINT('',(7.01759999912457,2.964,6.52800003889039));
#98313=CARTESIAN_POINT('',(7.0176,-4.08,6.528));
#98314=CARTESIAN_POINT('',(7.10945460790829,2.964,7.27219995625688));
#98315=CARTESIAN_POINT('Ctrl Pts',(7.10945460790824,2.964,7.27219995625657));
#98316=CARTESIAN_POINT('Ctrl Pts',(7.07010676471875,2.964,7.02501555776906));
#98317=CARTESIAN_POINT('Ctrl Pts',(7.0393340867141,2.964,6.77791646744438));
#98318=CARTESIAN_POINT('Ctrl Pts',(7.01759999655105,2.964,6.5280000391142));
#98319=CARTESIAN_POINT('',(7.1959607894463,2.8235504329007,7.74940308223601));
#98320=CARTESIAN_POINT('Ctrl Pts',(7.1959607894463,2.8235504329007,7.74940308223601));
#98321=CARTESIAN_POINT('Ctrl Pts',(7.16707443778447,2.91473432807616,7.60709256187426));
#98322=CARTESIAN_POINT('Ctrl Pts',(7.13617229126044,2.964,7.44004129019165));
#98323=CARTESIAN_POINT('Ctrl Pts',(7.10945460790829,2.964,7.27219995625688));
#98324=CARTESIAN_POINT('',(7.97548942358869,1.15565058469624,10.3765642386028));
#98325=CARTESIAN_POINT('Ctrl Pts',(7.97548942358869,1.15565058469624,10.3765642386028));
#98326=CARTESIAN_POINT('Ctrl Pts',(7.92841680860499,1.23817684922741,10.2451356716828));
#98327=CARTESIAN_POINT('Ctrl Pts',(7.88185377697889,1.32081047655035,10.1137894131233));
#98328=CARTESIAN_POINT('Ctrl Pts',(7.83611965044893,1.4035750711076,9.98250367791854));
#98329=CARTESIAN_POINT('Ctrl Pts',(7.78358181411942,1.49865227171574,9.83168701229214));
#98330=CARTESIAN_POINT('Ctrl Pts',(7.73213915445198,1.59390230515535,9.68094939752157));
#98331=CARTESIAN_POINT('Ctrl Pts',(7.68228607385709,1.68936095544672,9.53018191941683));
#98332=CARTESIAN_POINT('Ctrl Pts',(7.63343757783075,1.78289602777913,9.38245254207013));
#98333=CARTESIAN_POINT('Ctrl Pts',(7.58611766324347,1.87663139403831,9.23468984690772));
#98334=CARTESIAN_POINT('Ctrl Pts',(7.54077186667867,1.97060071830208,9.08676770712007));
#98335=CARTESIAN_POINT('Ctrl Pts',(7.50151579609986,2.05195040680673,8.95871081101122));
#98336=CARTESIAN_POINT('Ctrl Pts',(7.46373946462395,2.13347543389321,8.83053302698475));
#98337=CARTESIAN_POINT('Ctrl Pts',(7.42769958251337,2.2151976407413,8.70217698826003));
#98338=CARTESIAN_POINT('Ctrl Pts',(7.39230419049043,2.29545843458885,8.5761163009572));
#98339=CARTESIAN_POINT('Ctrl Pts',(7.35858386467001,2.37590941904463,8.44988328475345));
#98340=CARTESIAN_POINT('Ctrl Pts',(7.32674606854267,2.45657128438007,8.3234586653794));
#98341=CARTESIAN_POINT('Ctrl Pts',(7.29405805691174,2.53938719229378,8.1936579275392));
#98342=CARTESIAN_POINT('Ctrl Pts',(7.26335447294836,2.62242539445146,8.06365535232646));
#98343=CARTESIAN_POINT('Ctrl Pts',(7.23482034813647,2.70570828335953,7.93346923864727));
#98344=CARTESIAN_POINT('Ctrl Pts',(7.22138097542936,2.74493394006146,7.87215249196028));
#98345=CARTESIAN_POINT('Ctrl Pts',(7.20842230574121,2.78421387670058,7.81079556575853));
#98346=CARTESIAN_POINT('Ctrl Pts',(7.1959607894463,2.8235504329007,7.74940308223601));
#98347=CARTESIAN_POINT('Ctrl Pts',(8.26785692826664,0.924,11.1826993255823));
#98348=CARTESIAN_POINT('Ctrl Pts',(8.16503869361036,0.924000000000001,10.900623385729));
#98349=CARTESIAN_POINT('Ctrl Pts',(8.06230591927477,1.00344656775053,10.6189592620572));
#98350=CARTESIAN_POINT('Ctrl Pts',(7.97548942358868,1.15565058469624,10.3765642386028));
#98351=CARTESIAN_POINT('Ctrl Pts',(12.348,0.408,42.037449321013));
#98352=CARTESIAN_POINT('Ctrl Pts',(12.3293356677322,0.408,41.8347441976619));
#98353=CARTESIAN_POINT('Ctrl Pts',(12.2491547332484,0.408,41.431777240383));
#98354=CARTESIAN_POINT('Ctrl Pts',(11.9515727626208,0.408,40.6719616755841));
#98355=CARTESIAN_POINT('Ctrl Pts',(11.4307610148928,0.408,39.8019086889107));
#98356=CARTESIAN_POINT('Ctrl Pts',(10.8841273859392,0.408,38.7014536362885));
#98357=CARTESIAN_POINT('Ctrl Pts',(10.7053425599407,0.408,37.474766830819));
#98358=CARTESIAN_POINT('Ctrl Pts',(10.9975978291513,0.408,36.2617575584325));
#98359=CARTESIAN_POINT('Ctrl Pts',(11.762395791144,0.408,35.2772961441942));
#98360=CARTESIAN_POINT('Ctrl Pts',(12.7774343330734,0.408,34.5940530264168));
#98361=CARTESIAN_POINT('Ctrl Pts',(13.6438993253844,0.408,34.0639119954373));
#98362=CARTESIAN_POINT('Ctrl Pts',(14.2563720009146,0.408,33.5240486245267));
#98363=CARTESIAN_POINT('Ctrl Pts',(14.6230727172179,0.408,33.0266397369592));
#98364=CARTESIAN_POINT('Ctrl Pts',(14.7520512685869,0.408,32.5233081857418));
#98365=CARTESIAN_POINT('Ctrl Pts',(14.72627612058,0.408,32.1151402003716));
#98366=CARTESIAN_POINT('Ctrl Pts',(14.5982512199706,0.408,31.5160291164143));
#98367=CARTESIAN_POINT('Ctrl Pts',(14.1926078528925,0.408,30.6420288149888));
#98368=CARTESIAN_POINT('Ctrl Pts',(13.5644842062294,0.408,29.1492480693531));
#98369=CARTESIAN_POINT('Ctrl Pts',(13.1029533106643,0.408,27.6651812531195));
#98370=CARTESIAN_POINT('Ctrl Pts',(12.6560033050097,0.408,26.0711413023541));
#98371=CARTESIAN_POINT('Ctrl Pts',(12.2193900748355,0.408,24.4678689044597));
#98372=CARTESIAN_POINT('Ctrl Pts',(11.6714124934966,0.408,22.4795644823352));
#98373=CARTESIAN_POINT('Ctrl Pts',(10.7256257418815,0.408,19.4196973710059));
#98374=CARTESIAN_POINT('Ctrl Pts',(9.73067490339078,0.408,16.4328440977713));
#98375=CARTESIAN_POINT('Ctrl Pts',(8.71690211803928,0.408,13.294725251134));
#98376=CARTESIAN_POINT('Ctrl Pts',(8.14529762208715,0.408,11.7237141318561));
#98377=CARTESIAN_POINT('Ctrl Pts',(7.86706805722616,0.408,10.9590385811275));
#98378=CARTESIAN_POINT('Ctrl Pts',(12.4262089865968,0.408,42.0302481290153));
#98379=CARTESIAN_POINT('Ctrl Pts',(12.407041514443,0.408,41.8222299675208));
#98380=CARTESIAN_POINT('Ctrl Pts',(12.3247745295799,0.408,41.4088555280366));
#98381=CARTESIAN_POINT('Ctrl Pts',(12.0211738664984,0.408,40.6349151774764));
#98382=CARTESIAN_POINT('Ctrl Pts',(11.4975746041849,0.408,39.7608196137453));
#98383=CARTESIAN_POINT('Ctrl Pts',(10.9598179347726,0.408,38.675714715495));
#98384=CARTESIAN_POINT('Ctrl Pts',(10.7857556730067,0.408,37.4782170679473));
#98385=CARTESIAN_POINT('Ctrl Pts',(11.0708840374197,0.408,36.2963924897708));
#98386=CARTESIAN_POINT('Ctrl Pts',(11.8144929812671,0.408,35.3380422741074));
#98387=CARTESIAN_POINT('Ctrl Pts',(12.8166027375096,0.408,34.6616909757881));
#98388=CARTESIAN_POINT('Ctrl Pts',(13.6886183136859,0.408,34.1291779206297));
#98389=CARTESIAN_POINT('Ctrl Pts',(14.3134155906142,0.408,33.5785454640157));
#98390=CARTESIAN_POINT('Ctrl Pts',(14.6948792272124,0.408,33.0635168942324));
#98391=CARTESIAN_POINT('Ctrl Pts',(14.8316844100114,0.408,32.5308695841929));
#98392=CARTESIAN_POINT('Ctrl Pts',(14.804346338616,0.408,32.1037914102775));
#98393=CARTESIAN_POINT('Ctrl Pts',(14.6715776101179,0.408,31.4862764667729));
#98394=CARTESIAN_POINT('Ctrl Pts',(14.2634371814432,0.408,30.6086052959154));
#98395=CARTESIAN_POINT('Ctrl Pts',(13.6389720109982,0.408,29.1233338664017));
#98396=CARTESIAN_POINT('Ctrl Pts',(13.178243006681,0.408,27.6432224346962));
#98397=CARTESIAN_POINT('Ctrl Pts',(12.7317968740594,0.408,26.0503759497634));
#98398=CARTESIAN_POINT('Ctrl Pts',(12.2951426945594,0.408,24.4472662518418));
#98399=CARTESIAN_POINT('Ctrl Pts',(11.7469042071722,0.408,22.4577846978806));
#98400=CARTESIAN_POINT('Ctrl Pts',(10.8000742806557,0.408,19.3946624048871));
#98401=CARTESIAN_POINT('Ctrl Pts',(9.80548641546268,0.407999999999999,16.4089323484146));
#98402=CARTESIAN_POINT('Ctrl Pts',(8.79135149928353,0.408000000000001,13.2696900665871));
#98403=CARTESIAN_POINT('Ctrl Pts',(8.21899977033033,0.407999999999999,11.6965458507707));
#98404=CARTESIAN_POINT('Ctrl Pts',(7.94087412135137,0.408,10.9321840163567));
#98405=CARTESIAN_POINT('Ctrl Pts',(12.581955104232,0.473055248537292,42.0159076069757));
#98406=CARTESIAN_POINT('Ctrl Pts',(12.5618055796328,0.473055248537293,41.7971742246958));
#98407=CARTESIAN_POINT('Ctrl Pts',(12.4753204441731,0.473055248537293,41.3633235477922));
#98408=CARTESIAN_POINT('Ctrl Pts',(12.1597821186542,0.473055248537292,40.5609508438889));
#98409=CARTESIAN_POINT('Ctrl Pts',(11.6306919845739,0.473055248537292,39.6791381576489));
#98410=CARTESIAN_POINT('Ctrl Pts',(11.1105229237936,0.473055248537292,38.6243202097953));
#98411=CARTESIAN_POINT('Ctrl Pts',(10.9458889057599,0.473055248537292,37.4851605747719));
#98412=CARTESIAN_POINT('Ctrl Pts',(11.2168938631936,0.473055248537292,36.3652890517585));
#98413=CARTESIAN_POINT('Ctrl Pts',(11.9180174414507,0.473055248537292,35.4590386817689));
#98414=CARTESIAN_POINT('Ctrl Pts',(12.8946520834261,0.473055248537292,34.796515348691));
#98415=CARTESIAN_POINT('Ctrl Pts',(13.7775240669142,0.473055248537292,34.2591964757362));
#98416=CARTESIAN_POINT('Ctrl Pts',(14.4271163836494,0.473055248537292,33.6868645901221));
#98417=CARTESIAN_POINT('Ctrl Pts',(14.8379372503615,0.473055248537292,33.1372592611523));
#98418=CARTESIAN_POINT('Ctrl Pts',(14.9902008053167,0.473055248537292,32.5457514490063));
#98419=CARTESIAN_POINT('Ctrl Pts',(14.9595880150098,0.473055248537292,32.0813605528424));
#98420=CARTESIAN_POINT('Ctrl Pts',(14.8180716457112,0.473055248537292,31.4267941892507));
#98421=CARTESIAN_POINT('Ctrl Pts',(14.404321342134,0.473055248537292,30.5421242336123));
#98422=CARTESIAN_POINT('Ctrl Pts',(13.7875862672428,0.473055248537292,29.0715350395797));
#98423=CARTESIAN_POINT('Ctrl Pts',(13.3281948697516,0.473055248537292,27.5994860312853));
#98424=CARTESIAN_POINT('Ctrl Pts',(12.8827146686647,0.473055248537292,26.0089895623799));
#98425=CARTESIAN_POINT('Ctrl Pts',(12.4460283648194,0.473055248537292,24.4062796267624));
#98426=CARTESIAN_POINT('Ctrl Pts',(11.897212710331,0.473055248537292,22.4143751808534));
#98427=CARTESIAN_POINT('Ctrl Pts',(10.9483274733356,0.473055248537292,19.3447813493081));
#98428=CARTESIAN_POINT('Ctrl Pts',(9.95449421874235,0.473055248537291,16.3614278429735));
#98429=CARTESIAN_POINT('Ctrl Pts',(8.93959102601856,0.473055248537292,13.2197414791673));
#98430=CARTESIAN_POINT('Ctrl Pts',(8.36577664166789,0.473055248537291,11.6425235888116));
#98431=CARTESIAN_POINT('Ctrl Pts',(8.08785221741985,0.473055248537292,10.8787055813861));
#98432=CARTESIAN_POINT('Ctrl Pts',(12.646736323466,0.629460183660257,42.0099427937509));
#98433=CARTESIAN_POINT('Ctrl Pts',(12.626182924755,0.629460183660258,41.7867213486322));
#98434=CARTESIAN_POINT('Ctrl Pts',(12.5379284974733,0.629460183660258,41.3444114032542));
#98435=CARTESIAN_POINT('Ctrl Pts',(12.2174359085071,0.629460183660257,40.5301422030716));
#98436=CARTESIAN_POINT('Ctrl Pts',(11.6860758153009,0.629460183660256,39.6451967054032));
#98437=CARTESIAN_POINT('Ctrl Pts',(11.1732013451346,0.629460183660256,38.6029112675029));
#98438=CARTESIAN_POINT('Ctrl Pts',(11.0124943973279,0.629460183660256,37.4880654661885));
#98439=CARTESIAN_POINT('Ctrl Pts',(11.2776408422597,0.629460183660255,36.3939284497855));
#98440=CARTESIAN_POINT('Ctrl Pts',(11.9610261122155,0.629460183660255,35.5093720750203));
#98441=CARTESIAN_POINT('Ctrl Pts',(12.9271273497437,0.629460183660255,34.8526242972181));
#98442=CARTESIAN_POINT('Ctrl Pts',(13.8144693967793,0.629460183660255,34.3132874952525));
#98443=CARTESIAN_POINT('Ctrl Pts',(14.4744331847702,0.629460183660255,33.7318712545294));
#98444=CARTESIAN_POINT('Ctrl Pts',(14.8974552701336,0.629460183660255,33.1680022242259));
#98445=CARTESIAN_POINT('Ctrl Pts',(15.0561190850721,0.629460183660255,32.5519007446637));
#98446=CARTESIAN_POINT('Ctrl Pts',(15.0241066822088,0.629460183660255,32.072069761124));
#98447=CARTESIAN_POINT('Ctrl Pts',(14.8791134736059,0.629460183660255,31.4019992941433));
#98448=CARTESIAN_POINT('Ctrl Pts',(14.4628824756264,0.629460183660255,30.5144902537932));
#98449=CARTESIAN_POINT('Ctrl Pts',(13.8494654471821,0.629460183660255,29.0499451471956));
#98450=CARTESIAN_POINT('Ctrl Pts',(13.3905704701645,0.629460183660255,27.5812925495815));
#98451=CARTESIAN_POINT('Ctrl Pts',(12.9454833732632,0.629460183660255,25.9917673847204));
#98452=CARTESIAN_POINT('Ctrl Pts',(12.5087951337059,0.629460183660255,24.3892412418576));
#98453=CARTESIAN_POINT('Ctrl Pts',(11.9597260958242,0.629460183660255,22.3963108112752));
#98454=CARTESIAN_POINT('Ctrl Pts',(11.0099910748761,0.629460183660255,19.3240277115474));
#98455=CARTESIAN_POINT('Ctrl Pts',(10.0164790416783,0.629460183660255,16.3416950229929));
#98456=CARTESIAN_POINT('Ctrl Pts',(9.00124539599189,0.629460183660255,13.1989442398348));
#98457=CARTESIAN_POINT('Ctrl Pts',(8.42682850339849,0.629460183660254,11.6200722130095));
#98458=CARTESIAN_POINT('Ctrl Pts',(8.14898645568258,0.629460183660255,10.8564616996591));
#98459=CARTESIAN_POINT('Ctrl Pts',(12.646736323466,0.708000000000003,42.0099427937509));
#98460=CARTESIAN_POINT('Ctrl Pts',(12.626182924755,0.708000000000003,41.7867213486322));
#98461=CARTESIAN_POINT('Ctrl Pts',(12.5379284974733,0.708000000000002,41.3444114032542));
#98462=CARTESIAN_POINT('Ctrl Pts',(12.2174359085071,0.708000000000002,40.5301422030716));
#98463=CARTESIAN_POINT('Ctrl Pts',(11.6860758153009,0.708000000000001,39.6451967054032));
#98464=CARTESIAN_POINT('Ctrl Pts',(11.1732013451346,0.708000000000001,38.6029112675029));
#98465=CARTESIAN_POINT('Ctrl Pts',(11.0124943973279,0.708,37.4880654661885));
#98466=CARTESIAN_POINT('Ctrl Pts',(11.2776408422597,0.708,36.3939284497855));
#98467=CARTESIAN_POINT('Ctrl Pts',(11.9610261122155,0.708,35.5093720750203));
#98468=CARTESIAN_POINT('Ctrl Pts',(12.9271273497437,0.708,34.8526242972181));
#98469=CARTESIAN_POINT('Ctrl Pts',(13.8144693967793,0.708,34.3132874952525));
#98470=CARTESIAN_POINT('Ctrl Pts',(14.4744331847702,0.708,33.7318712545294));
#98471=CARTESIAN_POINT('Ctrl Pts',(14.8974552701336,0.708,33.1680022242259));
#98472=CARTESIAN_POINT('Ctrl Pts',(15.0561190850721,0.708,32.5519007446637));
#98473=CARTESIAN_POINT('Ctrl Pts',(15.0241066822088,0.708,32.072069761124));
#98474=CARTESIAN_POINT('Ctrl Pts',(14.8791134736059,0.708,31.4019992941433));
#98475=CARTESIAN_POINT('Ctrl Pts',(14.4628824756264,0.708,30.5144902537932));
#98476=CARTESIAN_POINT('Ctrl Pts',(13.8494654471821,0.708,29.0499451471956));
#98477=CARTESIAN_POINT('Ctrl Pts',(13.3905704701645,0.708,27.5812925495815));
#98478=CARTESIAN_POINT('Ctrl Pts',(12.9454833732632,0.708,25.9917673847204));
#98479=CARTESIAN_POINT('Ctrl Pts',(12.5087951337059,0.708,24.3892412418576));
#98480=CARTESIAN_POINT('Ctrl Pts',(11.9597260958242,0.708,22.3963108112752));
#98481=CARTESIAN_POINT('Ctrl Pts',(11.0099910748761,0.708,19.3240277115474));
#98482=CARTESIAN_POINT('Ctrl Pts',(10.0164790416783,0.708,16.3416950229929));
#98483=CARTESIAN_POINT('Ctrl Pts',(9.00124539599189,0.708,13.1989442398348));
#98484=CARTESIAN_POINT('Ctrl Pts',(8.42682850339849,0.708,11.6200722130095));
#98485=CARTESIAN_POINT('Ctrl Pts',(8.14898645568258,0.708,10.8564616996591));
#98486=CARTESIAN_POINT('',(7.86706805722616,0.408,10.9590385811275));
#98487=CARTESIAN_POINT('Ctrl Pts',(12.348,0.408,42.037449321013));
#98488=CARTESIAN_POINT('Ctrl Pts',(12.3293356677322,0.408,41.8347441976619));
#98489=CARTESIAN_POINT('Ctrl Pts',(12.2491547332484,0.408,41.431777240383));
#98490=CARTESIAN_POINT('Ctrl Pts',(11.9515727626208,0.408,40.6719616755841));
#98491=CARTESIAN_POINT('Ctrl Pts',(11.4307610148928,0.408,39.8019086889107));
#98492=CARTESIAN_POINT('Ctrl Pts',(10.8841273859392,0.408,38.7014536362885));
#98493=CARTESIAN_POINT('Ctrl Pts',(10.7053425599407,0.408,37.474766830819));
#98494=CARTESIAN_POINT('Ctrl Pts',(10.9975978291513,0.408,36.2617575584325));
#98495=CARTESIAN_POINT('Ctrl Pts',(11.762395791144,0.408,35.2772961441942));
#98496=CARTESIAN_POINT('Ctrl Pts',(12.7774343330734,0.408,34.5940530264168));
#98497=CARTESIAN_POINT('Ctrl Pts',(13.6438993253844,0.408,34.0639119954373));
#98498=CARTESIAN_POINT('Ctrl Pts',(14.2563720009146,0.408,33.5240486245267));
#98499=CARTESIAN_POINT('Ctrl Pts',(14.6230727172179,0.408,33.0266397369592));
#98500=CARTESIAN_POINT('Ctrl Pts',(14.7520512685869,0.408,32.5233081857418));
#98501=CARTESIAN_POINT('Ctrl Pts',(14.72627612058,0.408,32.1151402003716));
#98502=CARTESIAN_POINT('Ctrl Pts',(14.5982512199706,0.408,31.5160291164143));
#98503=CARTESIAN_POINT('Ctrl Pts',(14.1926078528925,0.408,30.6420288149888));
#98504=CARTESIAN_POINT('Ctrl Pts',(13.5644842062294,0.408,29.1492480693531));
#98505=CARTESIAN_POINT('Ctrl Pts',(13.1029533106643,0.408,27.6651812531195));
#98506=CARTESIAN_POINT('Ctrl Pts',(12.6560033050097,0.408,26.0711413023541));
#98507=CARTESIAN_POINT('Ctrl Pts',(12.2193900748355,0.408,24.4678689044597));
#98508=CARTESIAN_POINT('Ctrl Pts',(11.6714124934966,0.408,22.4795644823352));
#98509=CARTESIAN_POINT('Ctrl Pts',(10.7256257418815,0.408,19.4196973710059));
#98510=CARTESIAN_POINT('Ctrl Pts',(9.73067490339078,0.408,16.4328440977713));
#98511=CARTESIAN_POINT('Ctrl Pts',(8.71690211803928,0.408,13.294725251134));
#98512=CARTESIAN_POINT('Ctrl Pts',(8.14529762208715,0.408,11.7237141318561));
#98513=CARTESIAN_POINT('Ctrl Pts',(7.86706805722616,0.408,10.9590385811275));
#98514=CARTESIAN_POINT('Origin',(7.86706805722616,0.708,10.9590385811275));
#98515=CARTESIAN_POINT('Origin',(0.,0.408,45.696));
#98516=CARTESIAN_POINT('',(-7.86706805722818,0.408,10.9590385811275));
#98517=CARTESIAN_POINT('Ctrl Pts',(-7.86706805722818,0.408,10.9590385811275));
#98518=CARTESIAN_POINT('Ctrl Pts',(-8.14529762208872,0.408,11.7237141318567));
#98519=CARTESIAN_POINT('Ctrl Pts',(-8.71704186979063,0.408,13.2944622451918));
#98520=CARTESIAN_POINT('Ctrl Pts',(-9.73047444441272,0.408,16.4333423355267));
#98521=CARTESIAN_POINT('Ctrl Pts',(-10.7261073804545,0.408,19.4185393496298));
#98522=CARTESIAN_POINT('Ctrl Pts',(-11.6714712785442,0.408,22.4801977909835));
#98523=CARTESIAN_POINT('Ctrl Pts',(-12.3283245256811,0.408,24.863229880916));
#98524=CARTESIAN_POINT('Ctrl Pts',(-12.8745412424139,0.408,26.8802191948613));
#98525=CARTESIAN_POINT('Ctrl Pts',(-13.2776635653459,0.408,28.2207382228647));
#98526=CARTESIAN_POINT('Ctrl Pts',(-13.5275915188378,0.408,28.9655691222892));
#98527=CARTESIAN_POINT('Ctrl Pts',(-13.7965168172222,0.408,29.7066451167418));
#98528=CARTESIAN_POINT('Ctrl Pts',(-14.1174916376575,0.408,30.4559864726176));
#98529=CARTESIAN_POINT('Ctrl Pts',(-14.4607164581972,0.408,31.2259562265925));
#98530=CARTESIAN_POINT('Ctrl Pts',(-14.6785938108899,0.408,31.8124084143345));
#98531=CARTESIAN_POINT('Ctrl Pts',(-14.758965754309,0.408,32.318839178772));
#98532=CARTESIAN_POINT('Ctrl Pts',(-14.7021471218213,0.408,32.7251838170679));
#98533=CARTESIAN_POINT('Ctrl Pts',(-14.5601534893954,0.408,33.1087788993748));
#98534=CARTESIAN_POINT('Ctrl Pts',(-14.2578487820426,0.408,33.5241316135338));
#98535=CARTESIAN_POINT('Ctrl Pts',(-13.6438437735972,0.408,34.0632940521152));
#98536=CARTESIAN_POINT('Ctrl Pts',(-12.7773832461027,0.408,34.5944195816753));
#98537=CARTESIAN_POINT('Ctrl Pts',(-11.7611413721559,0.408,35.2761453566851));
#98538=CARTESIAN_POINT('Ctrl Pts',(-10.9988226749202,0.408,36.2620634912197));
#98539=CARTESIAN_POINT('Ctrl Pts',(-10.7057193819818,0.408,37.4749048193445));
#98540=CARTESIAN_POINT('Ctrl Pts',(-10.8844352537976,0.408,38.7015205845166));
#98541=CARTESIAN_POINT('Ctrl Pts',(-11.4308693301032,0.408,39.8019474928579));
#98542=CARTESIAN_POINT('Ctrl Pts',(-11.9516179428138,0.408,40.6719746799563));
#98543=CARTESIAN_POINT('Ctrl Pts',(-12.2491730342286,0.408,41.4317865452711));
#98544=CARTESIAN_POINT('Ctrl Pts',(-12.3293356677362,0.408,41.8347441976576));
#98545=CARTESIAN_POINT('Ctrl Pts',(-12.348,0.408,42.03744932101));
#98546=CARTESIAN_POINT('',(0.,0.408,10.9590385811275));
#98547=CARTESIAN_POINT('',(6.528,0.408,40.832));
#98548=CARTESIAN_POINT('Origin',(6.528,0.408,42.432));
#98549=CARTESIAN_POINT('',(-6.528,0.408,40.832));
#98550=CARTESIAN_POINT('Origin',(-6.528,0.408,42.432));
#98551=CARTESIAN_POINT('Origin',(-12.3479078516845,0.708,42.0374535543929));
#98552=CARTESIAN_POINT('',(-12.6467363234665,0.924,42.0099427937539));
#98553=CARTESIAN_POINT('Origin',(-12.348,0.924000000000001,42.03744932101));
#98554=CARTESIAN_POINT('',(-12.6467363234665,0.708000000000001,42.0099427937538));
#98555=CARTESIAN_POINT('',(-12.6467363234665,0.924000000000001,42.0099427937538));
#98556=CARTESIAN_POINT('Origin',(-12.348,0.708,42.03744932101));
#98557=CARTESIAN_POINT('Origin',(-12.348,0.924,42.03744932101));
#98558=CARTESIAN_POINT('Origin',(-12.348,0.924,42.03744932101));
#98559=CARTESIAN_POINT('Origin',(-12.348,0.708,42.0374493210099));
#98560=CARTESIAN_POINT('Origin',(-12.348,0.708,42.0374493210099));
#98561=CARTESIAN_POINT('Ctrl Pts',(-7.86706805722818,0.408,10.9590385811275));
#98562=CARTESIAN_POINT('Ctrl Pts',(-8.14529762208872,0.408,11.7237141318567));
#98563=CARTESIAN_POINT('Ctrl Pts',(-8.71704186979063,0.408,13.2944622451918));
#98564=CARTESIAN_POINT('Ctrl Pts',(-9.73047444441272,0.408,16.4333423355267));
#98565=CARTESIAN_POINT('Ctrl Pts',(-10.7261073804545,0.408,19.4185393496298));
#98566=CARTESIAN_POINT('Ctrl Pts',(-11.6714712785442,0.408,22.4801977909835));
#98567=CARTESIAN_POINT('Ctrl Pts',(-12.3283245256811,0.408,24.863229880916));
#98568=CARTESIAN_POINT('Ctrl Pts',(-12.8745412424139,0.408,26.8802191948613));
#98569=CARTESIAN_POINT('Ctrl Pts',(-13.2776635653459,0.408,28.2207382228647));
#98570=CARTESIAN_POINT('Ctrl Pts',(-13.5275915188378,0.408,28.9655691222892));
#98571=CARTESIAN_POINT('Ctrl Pts',(-13.7965168172222,0.408,29.7066451167418));
#98572=CARTESIAN_POINT('Ctrl Pts',(-14.1174916376575,0.408,30.4559864726176));
#98573=CARTESIAN_POINT('Ctrl Pts',(-14.4607164581972,0.408,31.2259562265925));
#98574=CARTESIAN_POINT('Ctrl Pts',(-14.6785938108899,0.408,31.8124084143345));
#98575=CARTESIAN_POINT('Ctrl Pts',(-14.758965754309,0.408,32.318839178772));
#98576=CARTESIAN_POINT('Ctrl Pts',(-14.7021471218213,0.408,32.7251838170679));
#98577=CARTESIAN_POINT('Ctrl Pts',(-14.5601534893954,0.408,33.1087788993748));
#98578=CARTESIAN_POINT('Ctrl Pts',(-14.2578487820426,0.408,33.5241316135338));
#98579=CARTESIAN_POINT('Ctrl Pts',(-13.6438437735972,0.408,34.0632940521152));
#98580=CARTESIAN_POINT('Ctrl Pts',(-12.7773832461027,0.408,34.5944195816753));
#98581=CARTESIAN_POINT('Ctrl Pts',(-11.7611413721559,0.408,35.2761453566851));
#98582=CARTESIAN_POINT('Ctrl Pts',(-10.9988226749202,0.408,36.2620634912197));
#98583=CARTESIAN_POINT('Ctrl Pts',(-10.7057193819818,0.408,37.4749048193445));
#98584=CARTESIAN_POINT('Ctrl Pts',(-10.8844352537976,0.408,38.7015205845166));
#98585=CARTESIAN_POINT('Ctrl Pts',(-11.4308693301032,0.408,39.8019474928579));
#98586=CARTESIAN_POINT('Ctrl Pts',(-11.9516179428138,0.408,40.6719746799563));
#98587=CARTESIAN_POINT('Ctrl Pts',(-12.2491730342286,0.408,41.4317865452711));
#98588=CARTESIAN_POINT('Ctrl Pts',(-12.3293356677362,0.408,41.8347441976576));
#98589=CARTESIAN_POINT('Ctrl Pts',(-12.348,0.408,42.03744932101));
#98590=CARTESIAN_POINT('Ctrl Pts',(-7.9408741213534,0.408,10.9321840163568));
#98591=CARTESIAN_POINT('Ctrl Pts',(-8.21899448195459,0.408,11.6965386637911));
#98592=CARTESIAN_POINT('Ctrl Pts',(-8.79150002820804,0.408,13.2694389389543));
#98593=CARTESIAN_POINT('Ctrl Pts',(-9.80527206182065,0.408,16.4094120358171));
#98594=CARTESIAN_POINT('Ctrl Pts',(-10.8005761179624,0.408,19.3935296469743));
#98595=CARTESIAN_POINT('Ctrl Pts',(-11.7469489940788,0.408,22.4584202360245));
#98596=CARTESIAN_POINT('Ctrl Pts',(-12.4041693706504,0.408,24.8428586149106));
#98597=CARTESIAN_POINT('Ctrl Pts',(-12.9502306891845,0.408,26.8592184864153));
#98598=CARTESIAN_POINT('Ctrl Pts',(-13.3526242310787,0.408,28.1972479280124));
#98599=CARTESIAN_POINT('Ctrl Pts',(-13.6017477475719,0.408,28.9396772692248));
#98600=CARTESIAN_POINT('Ctrl Pts',(-13.8696691564005,0.408,29.6779559679235));
#98601=CARTESIAN_POINT('Ctrl Pts',(-14.188972446946,0.408,30.4233668377294));
#98602=CARTESIAN_POINT('Ctrl Pts',(-14.5329455827326,0.408,31.1951619690078));
#98603=CARTESIAN_POINT('Ctrl Pts',(-14.7542894776902,0.408,31.7898177864783));
#98604=CARTESIAN_POINT('Ctrl Pts',(-14.8386547730419,0.408,32.3155727527421));
#98605=CARTESIAN_POINT('Ctrl Pts',(-14.7789340688096,0.408,32.7447317667957));
#98606=CARTESIAN_POINT('Ctrl Pts',(-14.629183409932,0.408,33.1483645673388));
#98607=CARTESIAN_POINT('Ctrl Pts',(-14.3150723184658,0.408,33.5787328885495));
#98608=CARTESIAN_POINT('Ctrl Pts',(-13.6884615573532,0.408,34.1284959992061));
#98609=CARTESIAN_POINT('Ctrl Pts',(-12.816577976426,0.408,34.6620649760208));
#98610=CARTESIAN_POINT('Ctrl Pts',(-11.8132710691042,0.408,35.3369167701079));
#98611=CARTESIAN_POINT('Ctrl Pts',(-11.0721272704617,0.408,36.2967378483312));
#98612=CARTESIAN_POINT('Ctrl Pts',(-10.7861220821357,0.408,37.4783331896387));
#98613=CARTESIAN_POINT('Ctrl Pts',(-10.960131624409,0.408,38.6757938575208));
#98614=CARTESIAN_POINT('Ctrl Pts',(-11.4976792812224,0.408,39.7608508017226));
#98615=CARTESIAN_POINT('Ctrl Pts',(-12.0212210638666,0.408,40.6349324038072));
#98616=CARTESIAN_POINT('Ctrl Pts',(-12.3247915762225,0.408,41.4088622076599));
#98617=CARTESIAN_POINT('Ctrl Pts',(-12.407042265963,0.408,41.8222315403878));
#98618=CARTESIAN_POINT('Ctrl Pts',(-12.4262089865969,0.408,42.0302481290139));
#98619=CARTESIAN_POINT('Ctrl Pts',(-8.08785221742193,0.473055248537291,
10.8787055813863));
#98620=CARTESIAN_POINT('Ctrl Pts',(-8.36577308576392,0.473055248537292,
11.6425187562859));
#98621=CARTESIAN_POINT('Ctrl Pts',(-8.93974692360289,0.473055248537292,
13.2194998310699));
#98622=CARTESIAN_POINT('Ctrl Pts',(-9.95426584407475,0.473055248537292,
16.3618905475388));
#98623=CARTESIAN_POINT('Ctrl Pts',(-10.9488714128454,0.473055248537292,
19.343709455506));
#98624=CARTESIAN_POINT('Ctrl Pts',(-11.8972430237721,0.473055248537292,
22.4150157545571));
#98625=CARTESIAN_POINT('Ctrl Pts',(-12.5552259541882,0.473055248537292,
24.802337614812));
#98626=CARTESIAN_POINT('Ctrl Pts',(-13.1009715712584,0.473055248537292,
26.817426547811));
#98627=CARTESIAN_POINT('Ctrl Pts',(-13.5019423383403,0.473055248537292,
28.1505676628167));
#98628=CARTESIAN_POINT('Ctrl Pts',(-13.7494718765433,0.473055248537292,
28.8882437809313));
#98629=CARTESIAN_POINT('Ctrl Pts',(-14.0153723178963,0.473055248537292,
29.6208791675758));
#98630=CARTESIAN_POINT('Ctrl Pts',(-14.3312811591807,0.473055248537292,
30.3584027105315));
#98631=CARTESIAN_POINT('Ctrl Pts',(-14.6768487098997,0.473055248537292,
31.1339357497066));
#98632=CARTESIAN_POINT('Ctrl Pts',(-14.9049633344377,0.473055248537292,
31.7447250380521));
#98633=CARTESIAN_POINT('Ctrl Pts',(-14.9973884818485,0.473055248537292,
32.3092032034564));
#98634=CARTESIAN_POINT('Ctrl Pts',(-14.9317626077194,0.473055248537292,
32.7835254048073));
#98635=CARTESIAN_POINT('Ctrl Pts',(-14.7666231464089,0.473055248537292,
33.2271698211528));
#98636=CARTESIAN_POINT('Ctrl Pts',(-14.4292891563142,0.473055248537292,
33.6872556604146));
#98637=CARTESIAN_POINT('Ctrl Pts',(-13.7771527815462,0.473055248537292,
34.2582504768461));
#98638=CARTESIAN_POINT('Ctrl Pts',(-12.894911422127,0.473055248537292,34.7968855412878));
#98639=CARTESIAN_POINT('Ctrl Pts',(-11.9170146182718,0.473055248537292,
35.4579926075445));
#98640=CARTESIAN_POINT('Ctrl Pts',(-11.2178736627465,0.473055248537292,
36.365562487716));
#98641=CARTESIAN_POINT('Ctrl Pts',(-10.9461492507296,0.473055248537292,
37.4852260297065));
#98642=CARTESIAN_POINT('Ctrl Pts',(-11.1107671811473,0.473055248537292,
38.6243802726169));
#98643=CARTESIAN_POINT('Ctrl Pts',(-11.6307663593404,0.473055248537292,
39.6791570877032));
#98644=CARTESIAN_POINT('Ctrl Pts',(-12.1598187182913,0.473055248537292,
40.5609653170687));
#98645=CARTESIAN_POINT('Ctrl Pts',(-12.4753335077982,0.473055248537292,
41.3633294566678));
#98646=CARTESIAN_POINT('Ctrl Pts',(-12.5618060849566,0.473055248537292,
41.797175282291));
#98647=CARTESIAN_POINT('Ctrl Pts',(-12.5819551042324,0.473055248537292,
42.0159076069773));
#98648=CARTESIAN_POINT('Ctrl Pts',(-8.14898645568467,0.629460183660255,
10.8564616996593));
#98649=CARTESIAN_POINT('Ctrl Pts',(-8.42682850340027,0.629460183660255,
11.6200722130106));
#98650=CARTESIAN_POINT('Ctrl Pts',(-9.00140202108135,0.629460183660255,
13.1987032575008));
#98651=CARTESIAN_POINT('Ctrl Pts',(-10.0162479906236,0.629460183660255,
16.3421552779583));
#98652=CARTESIAN_POINT('Ctrl Pts',(-11.0105529606629,0.629460183660255,
19.3229835736891));
#98653=CARTESIAN_POINT('Ctrl Pts',(-11.9597534877299,0.629460183660255,
22.3969536172018));
#98654=CARTESIAN_POINT('Ctrl Pts',(-12.6180608664011,0.629460183660255,
24.7854940213506));
#98655=CARTESIAN_POINT('Ctrl Pts',(-13.1636737275955,0.629460183660255,
26.8000502819042));
#98656=CARTESIAN_POINT('Ctrl Pts',(-13.5640592992395,0.629460183660255,
28.1311741992264));
#98657=CARTESIAN_POINT('Ctrl Pts',(-13.8109276823942,0.629460183660255,
28.866880021582));
#98658=CARTESIAN_POINT('Ctrl Pts',(-14.0759824773703,0.629460183660255,
29.5971513030824));
#98659=CARTESIAN_POINT('Ctrl Pts',(-14.3904642268911,0.629460183660255,
30.3313802830276));
#98660=CARTESIAN_POINT('Ctrl Pts',(-14.7367190536345,0.629460183660255,
31.1084918464257));
#98661=CARTESIAN_POINT('Ctrl Pts',(-14.9676192527248,0.629460183660255,
31.7259447042262));
#98662=CARTESIAN_POINT('Ctrl Pts',(-15.0634216666442,0.629460183660255,
32.3065851128709));
#98663=CARTESIAN_POINT('Ctrl Pts',(-14.995310469097,0.629460183660255,32.799630218064));
#98664=CARTESIAN_POINT('Ctrl Pts',(-14.8237837226447,0.629460183660255,
33.2599421532119));
#98665=CARTESIAN_POINT('Ctrl Pts',(-14.4768570601396,0.629460183660255,
33.7323460288388));
#98666=CARTESIAN_POINT('Ctrl Pts',(-13.8140058769173,0.629460183660255,
34.312200058379));
#98667=CARTESIAN_POINT('Ctrl Pts',(-12.9275584185962,0.629460183660254,
34.852988598105));
#98668=CARTESIAN_POINT('Ctrl Pts',(-11.9601501028038,0.629460183660255,
35.5083657619793));
#98669=CARTESIAN_POINT('Ctrl Pts',(-11.2784416996154,0.629460183660255,
36.394137190602));
#98670=CARTESIAN_POINT('Ctrl Pts',(-11.0126908986932,0.629460183660255,
37.488108200426));
#98671=CARTESIAN_POINT('Ctrl Pts',(-11.1733979901704,0.629460183660255,
38.6029533695122));
#98672=CARTESIAN_POINT('Ctrl Pts',(-11.6861322554559,0.629460183660255,
39.6452112093278));
#98673=CARTESIAN_POINT('Ctrl Pts',(-12.2174647212886,0.629460183660255,
40.5301529508079));
#98674=CARTESIAN_POINT('Ctrl Pts',(-12.5379395610492,0.629460183660255,
41.3444180220226));
#98675=CARTESIAN_POINT('Ctrl Pts',(-12.6261829247595,0.629460183660255,
41.7867213486289));
#98676=CARTESIAN_POINT('Ctrl Pts',(-12.6467363234665,0.629460183660255,
42.0099427937538));
#98677=CARTESIAN_POINT('Ctrl Pts',(-8.14898645568467,0.708,10.8564616996593));
#98678=CARTESIAN_POINT('Ctrl Pts',(-8.42682850340027,0.708,11.6200722130106));
#98679=CARTESIAN_POINT('Ctrl Pts',(-9.00140202108135,0.708,13.1987032575008));
#98680=CARTESIAN_POINT('Ctrl Pts',(-10.0162479906236,0.708,16.3421552779583));
#98681=CARTESIAN_POINT('Ctrl Pts',(-11.0105529606629,0.708,19.3229835736891));
#98682=CARTESIAN_POINT('Ctrl Pts',(-11.9597534877299,0.708,22.3969536172018));
#98683=CARTESIAN_POINT('Ctrl Pts',(-12.6180608664011,0.708,24.7854940213506));
#98684=CARTESIAN_POINT('Ctrl Pts',(-13.1636737275955,0.708,26.8000502819042));
#98685=CARTESIAN_POINT('Ctrl Pts',(-13.5640592992395,0.708,28.1311741992264));
#98686=CARTESIAN_POINT('Ctrl Pts',(-13.8109276823942,0.708,28.866880021582));
#98687=CARTESIAN_POINT('Ctrl Pts',(-14.0759824773703,0.708,29.5971513030824));
#98688=CARTESIAN_POINT('Ctrl Pts',(-14.3904642268911,0.708,30.3313802830276));
#98689=CARTESIAN_POINT('Ctrl Pts',(-14.7367190536345,0.708,31.1084918464257));
#98690=CARTESIAN_POINT('Ctrl Pts',(-14.9676192527248,0.708,31.7259447042262));
#98691=CARTESIAN_POINT('Ctrl Pts',(-15.0634216666442,0.708,32.3065851128709));
#98692=CARTESIAN_POINT('Ctrl Pts',(-14.995310469097,0.708,32.799630218064));
#98693=CARTESIAN_POINT('Ctrl Pts',(-14.8237837226447,0.708,33.2599421532119));
#98694=CARTESIAN_POINT('Ctrl Pts',(-14.4768570601396,0.708,33.7323460288388));
#98695=CARTESIAN_POINT('Ctrl Pts',(-13.8140058769173,0.708,34.312200058379));
#98696=CARTESIAN_POINT('Ctrl Pts',(-12.9275584185962,0.708,34.852988598105));
#98697=CARTESIAN_POINT('Ctrl Pts',(-11.9601501028038,0.708,35.5083657619793));
#98698=CARTESIAN_POINT('Ctrl Pts',(-11.2784416996154,0.708,36.394137190602));
#98699=CARTESIAN_POINT('Ctrl Pts',(-11.0126908986932,0.708,37.488108200426));
#98700=CARTESIAN_POINT('Ctrl Pts',(-11.1733979901704,0.708,38.6029533695122));
#98701=CARTESIAN_POINT('Ctrl Pts',(-11.6861322554559,0.708,39.6452112093278));
#98702=CARTESIAN_POINT('Ctrl Pts',(-12.2174647212886,0.708,40.5301529508079));
#98703=CARTESIAN_POINT('Ctrl Pts',(-12.5379395610492,0.708,41.3444180220226));
#98704=CARTESIAN_POINT('Ctrl Pts',(-12.6261829247595,0.708,41.7867213486289));
#98705=CARTESIAN_POINT('Ctrl Pts',(-12.6467363234665,0.708,42.0099427937538));
#98706=CARTESIAN_POINT('',(-8.14898645568467,0.708,10.8564616996593));
#98707=CARTESIAN_POINT('Ctrl Pts',(-12.6467363234665,0.708,42.0099427937538));
#98708=CARTESIAN_POINT('Ctrl Pts',(-12.6261829247595,0.708,41.7867213486289));
#98709=CARTESIAN_POINT('Ctrl Pts',(-12.5379395610492,0.708,41.3444180220226));
#98710=CARTESIAN_POINT('Ctrl Pts',(-12.2174647212886,0.708,40.5301529508079));
#98711=CARTESIAN_POINT('Ctrl Pts',(-11.6861322554559,0.708,39.6452112093278));
#98712=CARTESIAN_POINT('Ctrl Pts',(-11.1733979901704,0.708,38.6029533695122));
#98713=CARTESIAN_POINT('Ctrl Pts',(-11.0126908986932,0.708,37.488108200426));
#98714=CARTESIAN_POINT('Ctrl Pts',(-11.2784416996154,0.708,36.394137190602));
#98715=CARTESIAN_POINT('Ctrl Pts',(-11.9601501028038,0.708,35.5083657619793));
#98716=CARTESIAN_POINT('Ctrl Pts',(-12.9275584185962,0.708,34.852988598105));
#98717=CARTESIAN_POINT('Ctrl Pts',(-13.8140058769173,0.708,34.312200058379));
#98718=CARTESIAN_POINT('Ctrl Pts',(-14.4768570601396,0.708,33.7323460288388));
#98719=CARTESIAN_POINT('Ctrl Pts',(-14.8237837226447,0.708,33.2599421532119));
#98720=CARTESIAN_POINT('Ctrl Pts',(-14.995310469097,0.708,32.799630218064));
#98721=CARTESIAN_POINT('Ctrl Pts',(-15.0634216666442,0.708,32.3065851128709));
#98722=CARTESIAN_POINT('Ctrl Pts',(-14.9676192527248,0.708,31.7259447042262));
#98723=CARTESIAN_POINT('Ctrl Pts',(-14.7367190536345,0.708,31.1084918464257));
#98724=CARTESIAN_POINT('Ctrl Pts',(-14.3904642268911,0.708,30.3313802830276));
#98725=CARTESIAN_POINT('Ctrl Pts',(-14.0759824773703,0.708,29.5971513030824));
#98726=CARTESIAN_POINT('Ctrl Pts',(-13.8109276823942,0.708,28.866880021582));
#98727=CARTESIAN_POINT('Ctrl Pts',(-13.5640592992395,0.708,28.1311741992264));
#98728=CARTESIAN_POINT('Ctrl Pts',(-13.1636737275955,0.708,26.8000502819042));
#98729=CARTESIAN_POINT('Ctrl Pts',(-12.6180608664011,0.708,24.7854940213506));
#98730=CARTESIAN_POINT('Ctrl Pts',(-11.9597534877299,0.708,22.3969536172018));
#98731=CARTESIAN_POINT('Ctrl Pts',(-11.0105529606629,0.708,19.3229835736891));
#98732=CARTESIAN_POINT('Ctrl Pts',(-10.0162479906236,0.708,16.3421552779583));
#98733=CARTESIAN_POINT('Ctrl Pts',(-9.00140202108135,0.708,13.1987032575008));
#98734=CARTESIAN_POINT('Ctrl Pts',(-8.42682850340027,0.708,11.6200722130106));
#98735=CARTESIAN_POINT('Ctrl Pts',(-8.14898645568467,0.708,10.8564616996593));
#98736=CARTESIAN_POINT('Origin',(-7.86706805722818,0.708,10.9590385811275));
#98737=CARTESIAN_POINT('Ctrl Pts',(-7.0176,-4.08,6.528));
#98738=CARTESIAN_POINT('Ctrl Pts',(-7.0176,10.608,6.528));
#98739=CARTESIAN_POINT('Ctrl Pts',(-7.02630542760862,-4.08,6.62809945148413));
#98740=CARTESIAN_POINT('Ctrl Pts',(-7.02630542760862,10.608,6.62809945148413));
#98741=CARTESIAN_POINT('Ctrl Pts',(-7.04627094533223,-4.08,6.82892101239418));
#98742=CARTESIAN_POINT('Ctrl Pts',(-7.04627094533223,10.608,6.82892101239418));
#98743=CARTESIAN_POINT('Ctrl Pts',(-7.0838832606686,-4.08,7.13202122232862));
#98744=CARTESIAN_POINT('Ctrl Pts',(-7.0838832606686,10.608,7.13202122232862));
#98745=CARTESIAN_POINT('Ctrl Pts',(-7.14936655486467,-4.08,7.5398929237269));
#98746=CARTESIAN_POINT('Ctrl Pts',(-7.14936655486467,10.608,7.5398929237269));
#98747=CARTESIAN_POINT('Ctrl Pts',(-7.25661399291583,-4.08,8.05627564242548));
#98748=CARTESIAN_POINT('Ctrl Pts',(-7.25661399291583,10.608,8.05627564242548));
#98749=CARTESIAN_POINT('Ctrl Pts',(-7.38869925602642,-4.08,8.58014320427852));
#98750=CARTESIAN_POINT('Ctrl Pts',(-7.38869925602642,10.608,8.58014320427852));
#98751=CARTESIAN_POINT('Ctrl Pts',(-7.54448066029731,-4.08,9.11333934177059));
#98752=CARTESIAN_POINT('Ctrl Pts',(-7.54448066029731,10.608,9.11333934177059));
#98753=CARTESIAN_POINT('Ctrl Pts',(-7.72198141303516,-4.08,9.65899621296523));
#98754=CARTESIAN_POINT('Ctrl Pts',(-7.72198141303516,10.608,9.65899621296523));
#98755=CARTESIAN_POINT('Ctrl Pts',(-7.91830414508894,-4.08,10.2215845279079));
#98756=CARTESIAN_POINT('Ctrl Pts',(-7.91830414508894,10.608,10.2215845279079));
#98757=CARTESIAN_POINT('Ctrl Pts',(-8.13003837377838,-4.08,10.8059423149972));
#98758=CARTESIAN_POINT('Ctrl Pts',(-8.13003837377838,10.608,10.8059423149972));
#98759=CARTESIAN_POINT('Ctrl Pts',(-8.35357461247532,-4.08,11.4165038934416));
#98760=CARTESIAN_POINT('Ctrl Pts',(-8.35357461247532,10.608,11.4165038934416));
#98761=CARTESIAN_POINT('Ctrl Pts',(-8.58546625544539,-4.08,12.056408353432));
#98762=CARTESIAN_POINT('Ctrl Pts',(-8.58546625544539,10.608,12.056408353432));
#98763=CARTESIAN_POINT('Ctrl Pts',(-8.82274435252017,-4.08,12.7267521352155));
#98764=CARTESIAN_POINT('Ctrl Pts',(-8.82274435252017,10.608,12.7267521352155));
#98765=CARTESIAN_POINT('Ctrl Pts',(-9.06332174046713,-4.08,13.4255332425537));
#98766=CARTESIAN_POINT('Ctrl Pts',(-9.06332174046713,10.608,13.4255332425537));
#98767=CARTESIAN_POINT('Ctrl Pts',(-9.3059347889759,-4.08,14.1482310979449));
#98768=CARTESIAN_POINT('Ctrl Pts',(-9.3059347889759,10.608,14.1482310979449));
#98769=CARTESIAN_POINT('Ctrl Pts',(-9.54992705159325,-4.08,14.8889496618037));
#98770=CARTESIAN_POINT('Ctrl Pts',(-9.54992705159325,10.608,14.8889496618037));
#98771=CARTESIAN_POINT('Ctrl Pts',(-9.79508602811817,-4.08,15.6413708166808));
#98772=CARTESIAN_POINT('Ctrl Pts',(-9.79508602811817,10.608,15.6413708166808));
#98773=CARTESIAN_POINT('Ctrl Pts',(-10.0414581777666,-4.08,16.3997893456033));
#98774=CARTESIAN_POINT('Ctrl Pts',(-10.0414581777666,10.608,16.3997893456033));
#98775=CARTESIAN_POINT('Ctrl Pts',(-10.2891746222215,-4.08,17.1601046394451));
#98776=CARTESIAN_POINT('Ctrl Pts',(-10.2891746222215,10.608,17.1601046394451));
#98777=CARTESIAN_POINT('Ctrl Pts',(-10.5382704524098,-4.08,17.920853526763));
#98778=CARTESIAN_POINT('Ctrl Pts',(-10.5382704524098,10.608,17.920853526763));
#98779=CARTESIAN_POINT('Ctrl Pts',(-10.7885123454294,-4.08,18.6841717409417));
#98780=CARTESIAN_POINT('Ctrl Pts',(-10.7885123454294,10.608,18.6841717409417));
#98781=CARTESIAN_POINT('Ctrl Pts',(-11.0394491705041,-4.08,19.454441635642));
#98782=CARTESIAN_POINT('Ctrl Pts',(-11.0394491705041,10.608,19.454441635642));
#98783=CARTESIAN_POINT('Ctrl Pts',(-11.2904565074993,-4.08,20.2370106667962));
#98784=CARTESIAN_POINT('Ctrl Pts',(-11.2904565074993,10.608,20.2370106667962));
#98785=CARTESIAN_POINT('Ctrl Pts',(-11.5407830377124,-4.08,21.0368752434028));
#98786=CARTESIAN_POINT('Ctrl Pts',(-11.5407830377124,10.608,21.0368752434028));
#98787=CARTESIAN_POINT('Ctrl Pts',(-11.7895961018281,-4.08,21.8574023995577));
#98788=CARTESIAN_POINT('Ctrl Pts',(-11.7895961018281,10.608,21.8574023995577));
#98789=CARTESIAN_POINT('Ctrl Pts',(-12.0360270133741,-4.08,22.6989792594677));
#98790=CARTESIAN_POINT('Ctrl Pts',(-12.0360270133741,10.608,22.6989792594677));
#98791=CARTESIAN_POINT('Ctrl Pts',(-12.2792174635072,-4.08,23.5578155700236));
#98792=CARTESIAN_POINT('Ctrl Pts',(-12.2792174635072,10.608,23.5578155700236));
#98793=CARTESIAN_POINT('Ctrl Pts',(-12.5183627807975,-4.08,24.4243412707551));
#98794=CARTESIAN_POINT('Ctrl Pts',(-12.5183627807975,10.608,24.4243412707551));
#98795=CARTESIAN_POINT('Ctrl Pts',(-12.7527764582694,-4.08,25.2847489984795));
#98796=CARTESIAN_POINT('Ctrl Pts',(-12.7527764582694,10.608,25.2847489984795));
#98797=CARTESIAN_POINT('Ctrl Pts',(-12.9819542120743,-4.08,26.1231223827779));
#98798=CARTESIAN_POINT('Ctrl Pts',(-12.9819542120743,10.608,26.1231223827779));
#98799=CARTESIAN_POINT('Ctrl Pts',(-13.2056470980325,-4.08,26.9233802340012));
#98800=CARTESIAN_POINT('Ctrl Pts',(-13.2056470980325,10.608,26.9233802340012));
#98801=CARTESIAN_POINT('Ctrl Pts',(-13.4239120315545,-4.08,27.6712450999953));
#98802=CARTESIAN_POINT('Ctrl Pts',(-13.4239120315545,10.608,27.6712450999953));
#98803=CARTESIAN_POINT('Ctrl Pts',(-13.6372170146976,-4.08,28.356323880339));
#98804=CARTESIAN_POINT('Ctrl Pts',(-13.6372170146976,10.608,28.356323880339));
#98805=CARTESIAN_POINT('Ctrl Pts',(-13.8464193628061,-4.08,28.9738645264783));
#98806=CARTESIAN_POINT('Ctrl Pts',(-13.8464193628061,10.608,28.9738645264783));
#98807=CARTESIAN_POINT('Ctrl Pts',(-14.0530623083977,-4.08,29.5273742099472));
#98808=CARTESIAN_POINT('Ctrl Pts',(-14.0530623083977,10.608,29.5273742099472));
#98809=CARTESIAN_POINT('Ctrl Pts',(-14.2582197141431,-4.08,30.027253712516));
#98810=CARTESIAN_POINT('Ctrl Pts',(-14.2582197141431,10.608,30.027253712516));
#98811=CARTESIAN_POINT('Ctrl Pts',(-14.4606799971795,-4.08,30.487449167326));
#98812=CARTESIAN_POINT('Ctrl Pts',(-14.4606799971795,10.608,30.487449167326));
#98813=CARTESIAN_POINT('Ctrl Pts',(-14.6552019413825,-4.08,30.9226538837488));
#98814=CARTESIAN_POINT('Ctrl Pts',(-14.6552019413825,10.608,30.9226538837488));
#98815=CARTESIAN_POINT('Ctrl Pts',(-14.8310295566836,-4.08,31.3454571086889));
#98816=CARTESIAN_POINT('Ctrl Pts',(-14.8310295566836,10.608,31.3454571086889));
#98817=CARTESIAN_POINT('Ctrl Pts',(-14.9695221769896,-4.08,31.7630680429362));
#98818=CARTESIAN_POINT('Ctrl Pts',(-14.9695221769896,10.608,31.7630680429362));
#98819=CARTESIAN_POINT('Ctrl Pts',(-15.048097310419,-4.08,32.1776017680614));
#98820=CARTESIAN_POINT('Ctrl Pts',(-15.048097310419,10.608,32.1776017680614));
#98821=CARTESIAN_POINT('Ctrl Pts',(-15.0458732472955,-4.08,32.5872458409768));
#98822=CARTESIAN_POINT('Ctrl Pts',(-15.0458732472955,10.608,32.5872458409768));
#98823=CARTESIAN_POINT('Ctrl Pts',(-14.9484729279408,-4.08,32.9871564326141));
#98824=CARTESIAN_POINT('Ctrl Pts',(-14.9484729279408,10.608,32.9871564326141));
#98825=CARTESIAN_POINT('Ctrl Pts',(-14.7538514224946,-4.08,33.3703634670857));
#98826=CARTESIAN_POINT('Ctrl Pts',(-14.7538514224946,10.608,33.3703634670857));
#98827=CARTESIAN_POINT('Ctrl Pts',(-14.4705118919343,-4.08,33.7298729261475));
#98828=CARTESIAN_POINT('Ctrl Pts',(-14.4705118919343,10.608,33.7298729261475));
#98829=CARTESIAN_POINT('Ctrl Pts',(-14.1146548169613,-4.08,34.0610864824011));
#98830=CARTESIAN_POINT('Ctrl Pts',(-14.1146548169613,10.608,34.0610864824011));
#98831=CARTESIAN_POINT('Ctrl Pts',(-13.7077402642199,-4.08,34.3639065568129));
#98832=CARTESIAN_POINT('Ctrl Pts',(-13.7077402642199,10.608,34.3639065568129));
#98833=CARTESIAN_POINT('Ctrl Pts',(-13.2738213034502,-4.08,34.6454993802762));
#98834=CARTESIAN_POINT('Ctrl Pts',(-13.2738213034502,10.608,34.6454993802762));
#98835=CARTESIAN_POINT('Ctrl Pts',(-12.837485108751,-4.08,34.9181535900641));
#98836=CARTESIAN_POINT('Ctrl Pts',(-12.837485108751,10.608,34.9181535900641));
#98837=CARTESIAN_POINT('Ctrl Pts',(-12.4217894296783,-4.08,35.1961083216792));
#98838=CARTESIAN_POINT('Ctrl Pts',(-12.4217894296783,10.608,35.1961083216792));
#98839=CARTESIAN_POINT('Ctrl Pts',(-12.046351900761,-4.08,35.4928858294795));
#98840=CARTESIAN_POINT('Ctrl Pts',(-12.046351900761,10.608,35.4928858294795));
#98841=CARTESIAN_POINT('Ctrl Pts',(-11.7250208885935,-4.08,35.8180786547651));
#98842=CARTESIAN_POINT('Ctrl Pts',(-11.7250208885935,10.608,35.8180786547651));
#98843=CARTESIAN_POINT('Ctrl Pts',(-11.464839430663,-4.08,36.175427704157));
#98844=CARTESIAN_POINT('Ctrl Pts',(-11.464839430663,10.608,36.175427704157));
#98845=CARTESIAN_POINT('Ctrl Pts',(-11.268703490835,-4.08,36.5642101034686));
#98846=CARTESIAN_POINT('Ctrl Pts',(-11.268703490835,10.608,36.5642101034686));
#98847=CARTESIAN_POINT('Ctrl Pts',(-11.1371764695444,-4.08,36.980031199346));
#98848=CARTESIAN_POINT('Ctrl Pts',(-11.1371764695444,10.608,36.980031199346));
#98849=CARTESIAN_POINT('Ctrl Pts',(-11.0709679278875,-4.08,37.4158119460019));
#98850=CARTESIAN_POINT('Ctrl Pts',(-11.0709679278875,10.608,37.4158119460019));
#98851=CARTESIAN_POINT('Ctrl Pts',(-11.0720880317847,-4.08,37.8627943234178));
#98852=CARTESIAN_POINT('Ctrl Pts',(-11.0720880317847,10.608,37.8627943234178));
#98853=CARTESIAN_POINT('Ctrl Pts',(-11.1408514716218,-4.08,38.3120740300041));
#98854=CARTESIAN_POINT('Ctrl Pts',(-11.1408514716218,10.608,38.3120740300041));
#98855=CARTESIAN_POINT('Ctrl Pts',(-11.2737132025484,-4.08,38.755967364186));
#98856=CARTESIAN_POINT('Ctrl Pts',(-11.2737132025484,10.608,38.755967364186));
#98857=CARTESIAN_POINT('Ctrl Pts',(-11.4604343652129,-4.08,39.1895865074084));
#98858=CARTESIAN_POINT('Ctrl Pts',(-11.4604343652129,10.608,39.1895865074084));
#98859=CARTESIAN_POINT('Ctrl Pts',(-11.6825137471463,-4.08,39.6119151152234));
#98860=CARTESIAN_POINT('Ctrl Pts',(-11.6825137471463,10.608,39.6119151152234));
#98861=CARTESIAN_POINT('Ctrl Pts',(-11.9174888407557,-4.08,40.0243956758678));
#98862=CARTESIAN_POINT('Ctrl Pts',(-11.9174888407557,10.608,40.0243956758678));
#98863=CARTESIAN_POINT('Ctrl Pts',(-12.1425787135405,-4.08,40.4298136303268));
#98864=CARTESIAN_POINT('Ctrl Pts',(-12.1425787135405,10.608,40.4298136303268));
#98865=CARTESIAN_POINT('Ctrl Pts',(-12.3384198670367,-4.08,40.831110140755));
#98866=CARTESIAN_POINT('Ctrl Pts',(-12.3384198670367,10.608,40.831110140755));
#98867=CARTESIAN_POINT('Ctrl Pts',(-12.4931832123844,-4.08,41.2301191386975));
#98868=CARTESIAN_POINT('Ctrl Pts',(-12.4931832123844,10.608,41.2301191386975));
#98869=CARTESIAN_POINT('Ctrl Pts',(-12.5795001090599,-4.08,41.5482135599962));
#98870=CARTESIAN_POINT('Ctrl Pts',(-12.5795001090599,10.608,41.5482135599962));
#98871=CARTESIAN_POINT('Ctrl Pts',(-12.6222832973086,-4.08,41.7862967053278));
#98872=CARTESIAN_POINT('Ctrl Pts',(-12.6222832973086,10.608,41.7862967053278));
#98873=CARTESIAN_POINT('Ctrl Pts',(-12.6410531968159,-4.08,41.9448017311272));
#98874=CARTESIAN_POINT('Ctrl Pts',(-12.6410531968159,10.608,41.9448017311272));
#98875=CARTESIAN_POINT('Ctrl Pts',(-12.648,-4.08,42.024));
#98876=CARTESIAN_POINT('Ctrl Pts',(-12.648,10.608,42.024));
#98877=CARTESIAN_POINT('',(-8.26785692826842,0.924,11.1826993255826));
#98878=CARTESIAN_POINT('Ctrl Pts',(-8.26785692826842,0.924,11.1826993255826));
#98879=CARTESIAN_POINT('Ctrl Pts',(-8.54361306627396,0.924,11.9392205016032));
#98880=CARTESIAN_POINT('Ctrl Pts',(-9.09212599991816,0.924,13.4722442013831));
#98881=CARTESIAN_POINT('Ctrl Pts',(-10.0793574851517,0.924,16.5387499289064));
#98882=CARTESIAN_POINT('Ctrl Pts',(-11.0930194846002,0.924000000000001,
19.5704317186628));
#98883=CARTESIAN_POINT('Ctrl Pts',(-12.0379540421531,0.924,22.6694941250056));
#98884=CARTESIAN_POINT('Ctrl Pts',(-12.676785825845,0.924,25.0072588185284));
#98885=CARTESIAN_POINT('Ctrl Pts',(-13.3134204366261,0.924,27.3367371289618));
#98886=CARTESIAN_POINT('Ctrl Pts',(-13.8892654107988,0.924,29.1794300100813));
#98887=CARTESIAN_POINT('Ctrl Pts',(-14.4608280370914,0.924,30.4864933436934));
#98888=CARTESIAN_POINT('Ctrl Pts',(-14.7969073569086,0.924,31.255443467967));
#98889=CARTESIAN_POINT('Ctrl Pts',(-15.0048415747375,0.924,31.8645500407944));
#98890=CARTESIAN_POINT('Ctrl Pts',(-15.0761879359655,0.924,32.5848794176223));
#98891=CARTESIAN_POINT('Ctrl Pts',(-14.8238908844334,0.923999999999999,
33.2948194019013));
#98892=CARTESIAN_POINT('Ctrl Pts',(-14.3877781203166,0.924,33.8201146754649));
#98893=CARTESIAN_POINT('Ctrl Pts',(-13.8907462265714,0.924,34.2368869147185));
#98894=CARTESIAN_POINT('Ctrl Pts',(-13.3725424358171,0.924,34.5834843095939));
#98895=CARTESIAN_POINT('Ctrl Pts',(-12.6910734237184,0.924,35.0111461040952));
#98896=CARTESIAN_POINT('Ctrl Pts',(-11.9032876540853,0.924,35.5613424749907));
#98897=CARTESIAN_POINT('Ctrl Pts',(-11.2537874910971,0.924,36.4518523554272));
#98898=CARTESIAN_POINT('Ctrl Pts',(-11.0113749925991,0.924,37.5398403917748));
#98899=CARTESIAN_POINT('Ctrl Pts',(-11.1874609600943,0.924,38.6392410506538));
#98900=CARTESIAN_POINT('Ctrl Pts',(-11.6999497096383,0.924,39.6710971369163));
#98901=CARTESIAN_POINT('Ctrl Pts',(-12.3296022375865,0.924,40.7164504695946));
#98902=CARTESIAN_POINT('Ctrl Pts',(-12.6060713603138,0.924,41.5682984715533));
#98903=CARTESIAN_POINT('Ctrl Pts',(-12.6467363234665,0.924,42.0099427937538));
#98904=CARTESIAN_POINT('',(-7.97548942359086,1.15565058469624,10.3765642386027));
#98905=CARTESIAN_POINT('Ctrl Pts',(-7.97548942359086,1.15565058469624,10.3765642386027));
#98906=CARTESIAN_POINT('Ctrl Pts',(-8.06230799714572,1.0034429248949,10.6189650635473));
#98907=CARTESIAN_POINT('Ctrl Pts',(-8.16503623275751,0.92400000000006,10.9006166345145));
#98908=CARTESIAN_POINT('Ctrl Pts',(-8.2678569282683,0.924,11.1826993255823));
#98909=CARTESIAN_POINT('',(-7.19596078944639,2.8235504329007,7.74940308223659));
#98910=CARTESIAN_POINT('Ctrl Pts',(-7.19596078944639,2.8235504329007,7.74940308223659));
#98911=CARTESIAN_POINT('Ctrl Pts',(-7.22233262615032,2.74030396336476,7.8793256784926));
#98912=CARTESIAN_POINT('Ctrl Pts',(-7.25093335954429,2.65731106826831,8.00908682877084));
#98913=CARTESIAN_POINT('Ctrl Pts',(-7.28159746422587,2.5745495730776,8.13865166883888));
#98914=CARTESIAN_POINT('Ctrl Pts',(-7.31161939938325,2.49352127409596,8.26550315423493));
#98915=CARTESIAN_POINT('Ctrl Pts',(-7.34361926028415,2.41271478452361,8.39216624339057));
#98916=CARTESIAN_POINT('Ctrl Pts',(-7.3774062658177,2.33210929399645,8.5186423305201));
#98917=CARTESIAN_POINT('Ctrl Pts',(-7.41168327760693,2.25033479798993,8.6469526753149));
#98918=CARTESIAN_POINT('Ctrl Pts',(-7.4477997057716,2.16876717340375,8.77507050652281));
#98919=CARTESIAN_POINT('Ctrl Pts',(-7.48551767859797,2.08738469125336,8.90303614781032));
#98920=CARTESIAN_POINT('Ctrl Pts',(-7.52666669782826,1.9985991847143,9.04264228885072));
#98921=CARTESIAN_POINT('Ctrl Pts',(-7.5697219334645,1.91003403589183,9.18206778255516));
#98922=CARTESIAN_POINT('Ctrl Pts',(-7.61432732220447,1.82166103025293,9.32140797710534));
#98923=CARTESIAN_POINT('Ctrl Pts',(-7.6664953999531,1.71830468790771,9.48437281853242));
#98924=CARTESIAN_POINT('Ctrl Pts',(-7.72078165008511,1.61521116652034,9.64722711387514));
#98925=CARTESIAN_POINT('Ctrl Pts',(-7.77656785595829,1.5123353298502,9.81013231365598));
#98926=CARTESIAN_POINT('Ctrl Pts',(-7.82095433614413,1.43048182835304,9.93974837750305));
#98927=CARTESIAN_POINT('Ctrl Pts',(-7.8662889047216,1.34876613526015,10.0693975485112));
#98928=CARTESIAN_POINT('Ctrl Pts',(-7.9122593737334,1.26716551546311,10.1991238167179));
#98929=CARTESIAN_POINT('Ctrl Pts',(-7.93321343005476,1.22997068104352,10.2582550718213));
#98930=CARTESIAN_POINT('Ctrl Pts',(-7.9542997016531,1.19279975515514,10.3174017130308));
#98931=CARTESIAN_POINT('Ctrl Pts',(-7.97548942359086,1.15565058469625,10.3765642386027));
#98932=CARTESIAN_POINT('',(-7.10945460790939,2.964,7.27219995625739));
#98933=CARTESIAN_POINT('Ctrl Pts',(-7.10945460790939,2.964,7.27219995625739));
#98934=CARTESIAN_POINT('Ctrl Pts',(-7.13617164034088,2.964,7.44003720108978));
#98935=CARTESIAN_POINT('Ctrl Pts',(-7.16707514154032,2.91473210657155,7.60709602897267));
#98936=CARTESIAN_POINT('Ctrl Pts',(-7.19596078944639,2.8235504329007,7.74940308223659));
#98937=CARTESIAN_POINT('',(-7.01760000081282,2.964,6.52800003819785));
#98938=CARTESIAN_POINT('Ctrl Pts',(-7.01760000330315,2.964,6.52800003798128));
#98939=CARTESIAN_POINT('Ctrl Pts',(-7.02446531775896,2.964,6.60694092546319));
#98940=CARTESIAN_POINT('Ctrl Pts',(-7.03215675137159,2.964,6.68470062724588));
#98941=CARTESIAN_POINT('Ctrl Pts',(-7.04064330589647,2.964,6.76177920847414));
#98942=CARTESIAN_POINT('Ctrl Pts',(-7.04922558187721,2.964,6.83972717361903));
#98943=CARTESIAN_POINT('Ctrl Pts',(-7.05862115895179,2.964,6.91697853001615));
#98944=CARTESIAN_POINT('Ctrl Pts',(-7.06884967735363,2.964,6.99406426404567));
#98945=CARTESIAN_POINT('Ctrl Pts',(-7.07915808333351,2.964,7.07175205913145));
#98946=CARTESIAN_POINT('Ctrl Pts',(-7.09031256144649,2.964,7.1492715590365));
#98947=CARTESIAN_POINT('Ctrl Pts',(-7.10238379369393,2.964,7.22718103044211));
#98948=CARTESIAN_POINT('Ctrl Pts',(-7.10470640653238,2.964,7.24217150820068));
#98949=CARTESIAN_POINT('Ctrl Pts',(-7.10706310656637,2.964,7.25717646899493));
#98950=CARTESIAN_POINT('Ctrl Pts',(-7.10945460790939,2.964,7.27219995625739));
#98951=CARTESIAN_POINT('',(-7.0176,2.748,6.528));
#98952=CARTESIAN_POINT('',(-7.0176,-4.08,6.528));
#98953=CARTESIAN_POINT('',(-7.06369006012712,2.748,6.95461383265843));
#98954=CARTESIAN_POINT('Origin',(-17.3375887932806,2.748,5.62885644979173));
#98955=CARTESIAN_POINT('',(-7.19430053092012,2.51634941530375,7.74120895321998));
#98956=CARTESIAN_POINT('Ctrl Pts',(-7.19430053092012,2.51634941530376,7.74120895321997));
#98957=CARTESIAN_POINT('Ctrl Pts',(-7.18139423288357,2.5572388274877,7.67739535408007));
#98958=CARTESIAN_POINT('Ctrl Pts',(-7.16841680020877,2.59304356056116,7.61051677367225));
#98959=CARTESIAN_POINT('Ctrl Pts',(-7.15568446739969,2.62349886615165,7.54138656787107));
#98960=CARTESIAN_POINT('Ctrl Pts',(-7.14341508067495,2.65284682050636,7.47476992800986));
#98961=CARTESIAN_POINT('Ctrl Pts',(-7.1313737350991,2.67722728429196,7.40606237419146));
#98962=CARTESIAN_POINT('Ctrl Pts',(-7.11979834628682,2.69640335049437,7.33597973689174));
#98963=CARTESIAN_POINT('Ctrl Pts',(-7.10857994715557,2.71498801904542,7.26805847652209));
#98964=CARTESIAN_POINT('Ctrl Pts',(-7.0977993730232,2.72868435141184,7.1988456068992));
#98965=CARTESIAN_POINT('Ctrl Pts',(-7.08762578934646,2.73727669046519,7.12898188155835));
#98966=CARTESIAN_POINT('Ctrl Pts',(-7.07920950084515,2.74438486460243,7.07118580036135));
#98967=CARTESIAN_POINT('Ctrl Pts',(-7.0712078148154,2.748,7.01294410869989));
#98968=CARTESIAN_POINT('Ctrl Pts',(-7.06369006012712,2.748,6.95461383265843));
#98969=CARTESIAN_POINT('',(-7.97249537063732,0.848449567099298,10.3682028984961));
#98970=CARTESIAN_POINT('Ctrl Pts',(-7.97249537063731,0.848449567099298,
10.3682028984961));
#98971=CARTESIAN_POINT('Ctrl Pts',(-7.65957903289542,1.39732053099838,9.49414527429354));
#98972=CARTESIAN_POINT('Ctrl Pts',(-7.37274783895309,1.9509970957918,8.62351966308919));
#98973=CARTESIAN_POINT('Ctrl Pts',(-7.19430053092012,2.51634941530375,7.74120895321998));
#98974=CARTESIAN_POINT('Ctrl Pts',(-8.14898645568466,0.707999999999999,
10.8564616996593));
#98975=CARTESIAN_POINT('Ctrl Pts',(-8.12815013435031,0.707999999999999,
10.7991959468286));
#98976=CARTESIAN_POINT('Ctrl Pts',(-8.10733389973439,0.713424220187055,
10.7419087307375));
#98977=CARTESIAN_POINT('Ctrl Pts',(-8.08689701837362,0.724116204510082,
10.6855367371928));
#98978=CARTESIAN_POINT('Ctrl Pts',(-8.06554794403206,0.735285421776732,
10.6266485996279));
#98979=CARTESIAN_POINT('Ctrl Pts',(-8.04461331168835,0.752203147474417,
10.5687589560619));
#98980=CARTESIAN_POINT('Ctrl Pts',(-8.02447437612234,0.774691026458215,
10.5128836557502));
#98981=CARTESIAN_POINT('Ctrl Pts',(-8.00642490774828,0.794845729232223,
10.4628055638589));
#98982=CARTESIAN_POINT('Ctrl Pts',(-7.98901420075669,0.819474709872172,
10.414344335255));
#98983=CARTESIAN_POINT('Ctrl Pts',(-7.97249537063731,0.848449567099298,
10.3682028984961));
#98984=CARTESIAN_POINT('Ctrl Pts',(-12.348,1.224,42.03744932101));
#98985=CARTESIAN_POINT('Ctrl Pts',(-12.3110725606702,1.224,41.6363966051328));
#98986=CARTESIAN_POINT('Ctrl Pts',(-12.0609852952635,1.224,40.8549204601091));
#98987=CARTESIAN_POINT('Ctrl Pts',(-11.4450821737987,1.224,39.8274092249604));
#98988=CARTESIAN_POINT('Ctrl Pts',(-10.8997688026688,1.224,38.7409075676707));
#98989=CARTESIAN_POINT('Ctrl Pts',(-10.7043533514793,1.224,37.5315890187733));
#98990=CARTESIAN_POINT('Ctrl Pts',(-10.9709851394883,1.224,36.3263525491271));
#98991=CARTESIAN_POINT('Ctrl Pts',(-11.6986135266186,1.224,35.3339416136743));
#98992=CARTESIAN_POINT('Ctrl Pts',(-12.5309171577631,1.224,34.7574741120408));
#98993=CARTESIAN_POINT('Ctrl Pts',(-13.2114636130569,1.224,34.3298336160849));
#98994=CARTESIAN_POINT('Ctrl Pts',(-13.7131082734894,1.224,33.9932968374398));
#98995=CARTESIAN_POINT('Ctrl Pts',(-14.1769757204202,1.224,33.6048339401135));
#98996=CARTESIAN_POINT('Ctrl Pts',(-14.5620228329377,1.224,33.1340383684088));
#98997=CARTESIAN_POINT('Ctrl Pts',(-14.7683961662382,1.224,32.5514380647304));
#98998=CARTESIAN_POINT('Ctrl Pts',(-14.711659402932,1.224,31.939868704061));
#98999=CARTESIAN_POINT('Ctrl Pts',(-14.5189773065471,1.224,31.3678083420515));
#99000=CARTESIAN_POINT('Ctrl Pts',(-14.1888423807734,1.224,30.613847819264));
#99001=CARTESIAN_POINT('Ctrl Pts',(-13.6063457415431,1.224,29.2804450588471));
#99002=CARTESIAN_POINT('Ctrl Pts',(-13.0245909094872,1.224,27.4180026826501));
#99003=CARTESIAN_POINT('Ctrl Pts',(-12.3871316955906,1.224,25.0852094102837));
#99004=CARTESIAN_POINT('Ctrl Pts',(-11.7493811375928,1.224,22.7517028806517));
#99005=CARTESIAN_POINT('Ctrl Pts',(-10.8084555662763,1.224,19.6656582368069));
#99006=CARTESIAN_POINT('Ctrl Pts',(-9.79376320963301,1.224,16.6304717567395));
#99007=CARTESIAN_POINT('Ctrl Pts',(-8.80744652629141,1.224,13.5670274338247));
#99008=CARTESIAN_POINT('Ctrl Pts',(-8.26166260011136,1.224,12.0417095524852));
#99009=CARTESIAN_POINT('Ctrl Pts',(-7.98599766308436,1.224,11.2854385811275));
#99010=CARTESIAN_POINT('Ctrl Pts',(-12.4262089865969,1.224,42.0302481290138));
#99011=CARTESIAN_POINT('Ctrl Pts',(-12.3884597397384,1.224,41.6182718077793));
#99012=CARTESIAN_POINT('Ctrl Pts',(-12.1313110647987,1.224,40.8188312736214));
#99013=CARTESIAN_POINT('Ctrl Pts',(-11.5118493291914,1.224,39.7863371802633));
#99014=CARTESIAN_POINT('Ctrl Pts',(-10.9750998698324,1.224,38.7143350236826));
#99015=CARTESIAN_POINT('Ctrl Pts',(-10.7847684351755,1.224,37.5336806373346));
#99016=CARTESIAN_POINT('Ctrl Pts',(-11.0449682137518,1.224,36.3591917863843));
#99017=CARTESIAN_POINT('Ctrl Pts',(-11.7523600195699,1.224,35.3934310919955));
#99018=CARTESIAN_POINT('Ctrl Pts',(-12.5726728148048,1.224,34.8237749281237));
#99019=CARTESIAN_POINT('Ctrl Pts',(-13.2536375709064,1.224,34.3961247440975));
#99020=CARTESIAN_POINT('Ctrl Pts',(-13.7595078804483,1.224,34.0569555347383));
#99021=CARTESIAN_POINT('Ctrl Pts',(-14.2321163943034,1.224,33.6610389297134));
#99022=CARTESIAN_POINT('Ctrl Pts',(-14.6305352247796,1.224,33.1760304630879));
#99023=CARTESIAN_POINT('Ctrl Pts',(-14.8490560326206,1.224,32.5605118065707));
#99024=CARTESIAN_POINT('Ctrl Pts',(-14.7884740076186,1.224,31.9202106499033));
#99025=CARTESIAN_POINT('Ctrl Pts',(-14.5917916222844,1.224,31.3385534447848));
#99026=CARTESIAN_POINT('Ctrl Pts',(-14.2600864674804,1.224,30.5805368096967));
#99027=CARTESIAN_POINT('Ctrl Pts',(-13.6804549117615,1.224,29.2541245480614));
#99028=CARTESIAN_POINT('Ctrl Pts',(-13.1002241344054,1.224,27.3967600289198));
#99029=CARTESIAN_POINT('Ctrl Pts',(-12.4629663663438,1.224,25.0648149363375));
#99030=CARTESIAN_POINT('Ctrl Pts',(-11.8249399914061,1.224,22.7302062906546));
#99031=CARTESIAN_POINT('Ctrl Pts',(-10.8829597173486,1.224,19.6407501735903));
#99032=CARTESIAN_POINT('Ctrl Pts',(-9.86851299468442,1.224,16.6063977618495));
#99033=CARTESIAN_POINT('Ctrl Pts',(-8.88199052732757,1.224,13.5422656081676));
#99034=CARTESIAN_POINT('Ctrl Pts',(-8.33547603090265,1.224,12.014852000593));
#99035=CARTESIAN_POINT('Ctrl Pts',(-8.05978824615506,1.224,11.2585415069229));
#99036=CARTESIAN_POINT('Ctrl Pts',(-12.5819547309417,1.15894437659295,42.0159076413485));
#99037=CARTESIAN_POINT('Ctrl Pts',(-12.5422059135609,1.15894437659295,41.5828655760323));
#99038=CARTESIAN_POINT('Ctrl Pts',(-12.2713534566526,1.15894437659295,40.7465873386517));
#99039=CARTESIAN_POINT('Ctrl Pts',(-11.6447101463389,1.15894437659295,39.7048928283908));
#99040=CARTESIAN_POINT('Ctrl Pts',(-11.1250833790616,1.15894437659295,38.661317107898));
#99041=CARTESIAN_POINT('Ctrl Pts',(-10.9448216674133,1.15894437659295,37.5380048122601));
#99042=CARTESIAN_POINT('Ctrl Pts',(-11.1924245222642,1.15894437659295,36.4246263108199));
#99043=CARTESIAN_POINT('Ctrl Pts',(-11.8590135202287,1.15894437659295,35.5120005020376));
#99044=CARTESIAN_POINT('Ctrl Pts',(-12.6562264341236,1.15894437659295,34.9560623847726));
#99045=CARTESIAN_POINT('Ctrl Pts',(-13.3376146000376,1.15894437659295,34.528402435818));
#99046=CARTESIAN_POINT('Ctrl Pts',(-13.8521536514053,1.15894437659294,34.1839876724815));
#99047=CARTESIAN_POINT('Ctrl Pts',(-14.3420333075769,1.15894437659295,33.7733258205512));
#99048=CARTESIAN_POINT('Ctrl Pts',(-14.7670742413869,1.15894437659295,33.2598860740197));
#99049=CARTESIAN_POINT('Ctrl Pts',(-15.0094967148898,1.15894437659295,32.5778425903243));
#99050=CARTESIAN_POINT('Ctrl Pts',(-14.9413046656758,1.15894437659295,31.8809237312434));
#99051=CARTESIAN_POINT('Ctrl Pts',(-14.736672983979,1.15894437659295,31.27991937865));
#99052=CARTESIAN_POINT('Ctrl Pts',(-14.4018732837384,1.15894437659295,30.5141308692897));
#99053=CARTESIAN_POINT('Ctrl Pts',(-13.8279413241913,1.15894437659295,29.2014197421003));
#99054=CARTESIAN_POINT('Ctrl Pts',(-13.2507991784978,1.15894437659295,27.3543817300241));
#99055=CARTESIAN_POINT('Ctrl Pts',(-12.6139760164723,1.15894437659295,25.0241712948571));
#99056=CARTESIAN_POINT('Ctrl Pts',(-11.9753835861599,1.15894437659295,22.6873385363609));
#99057=CARTESIAN_POINT('Ctrl Pts',(-11.0313149108527,1.15894437659295,19.5910967451308));
#99058=CARTESIAN_POINT('Ctrl Pts',(-10.0174132153215,1.15894437659295,16.5585986749172));
#99059=CARTESIAN_POINT('Ctrl Pts',(-9.03040284012067,1.15894437659295,13.4928334566676));
#99060=CARTESIAN_POINT('Ctrl Pts',(-8.48247082810459,1.15894437659295,11.9614279444147));
#99061=CARTESIAN_POINT('Ctrl Pts',(-8.20673516090307,1.15894437659295,11.2049785466421));
#99062=CARTESIAN_POINT('Ctrl Pts',(-12.6467363234665,1.00253981633974,42.0099427937538));
#99063=CARTESIAN_POINT('Ctrl Pts',(-12.6060713603138,1.00253981633975,41.5682984715533));
#99064=CARTESIAN_POINT('Ctrl Pts',(-12.3296022375865,1.00253981633974,40.7164504695946));
#99065=CARTESIAN_POINT('Ctrl Pts',(-11.6999497096383,1.00253981633974,39.6710971369163));
#99066=CARTESIAN_POINT('Ctrl Pts',(-11.1874609600943,1.00253981633974,38.6392410506538));
#99067=CARTESIAN_POINT('Ctrl Pts',(-11.0113749925991,1.00253981633974,37.5398403917748));
#99068=CARTESIAN_POINT('Ctrl Pts',(-11.2537874910971,1.00253981633974,36.4518523554272));
#99069=CARTESIAN_POINT('Ctrl Pts',(-11.9032876540853,1.00253981633974,35.5613424749907));
#99070=CARTESIAN_POINT('Ctrl Pts',(-12.6910734237184,1.00253981633974,35.0111461040952));
#99071=CARTESIAN_POINT('Ctrl Pts',(-13.3725424358171,1.00253981633974,34.5834843095939));
#99072=CARTESIAN_POINT('Ctrl Pts',(-13.8907462265714,1.00253981633974,34.2368869147185));
#99073=CARTESIAN_POINT('Ctrl Pts',(-14.3877781203166,1.00253981633974,33.8201146754649));
#99074=CARTESIAN_POINT('Ctrl Pts',(-14.8238908844334,1.00253981633974,33.2948194019013));
#99075=CARTESIAN_POINT('Ctrl Pts',(-15.0761879359655,1.00253981633974,32.5848794176223));
#99076=CARTESIAN_POINT('Ctrl Pts',(-15.0048415747375,1.00253981633974,31.8645500407944));
#99077=CARTESIAN_POINT('Ctrl Pts',(-14.7969073569086,1.00253981633974,31.255443467967));
#99078=CARTESIAN_POINT('Ctrl Pts',(-14.4608280370914,1.00253981633974,30.4864933436934));
#99079=CARTESIAN_POINT('Ctrl Pts',(-13.8892654107988,1.00253981633974,29.1794300100813));
#99080=CARTESIAN_POINT('Ctrl Pts',(-13.3134204366261,1.00253981633974,27.3367371289618));
#99081=CARTESIAN_POINT('Ctrl Pts',(-12.676785825845,1.00253981633974,25.0072588185284));
#99082=CARTESIAN_POINT('Ctrl Pts',(-12.0379540421531,1.00253981633974,22.6694941250056));
#99083=CARTESIAN_POINT('Ctrl Pts',(-11.0930194846002,1.00253981633975,19.5704317186628));
#99084=CARTESIAN_POINT('Ctrl Pts',(-10.0793574851517,1.00253981633975,16.5387499289064));
#99085=CARTESIAN_POINT('Ctrl Pts',(-9.09212599991816,1.00253981633974,13.4722442013831));
#99086=CARTESIAN_POINT('Ctrl Pts',(-8.54361306627396,1.00253981633975,11.9392205016032));
#99087=CARTESIAN_POINT('Ctrl Pts',(-8.26785692826842,1.00253981633974,11.1826993255826));
#99088=CARTESIAN_POINT('Ctrl Pts',(-12.6467363234665,0.924,42.0099427937538));
#99089=CARTESIAN_POINT('Ctrl Pts',(-12.6060713603138,0.924,41.5682984715533));
#99090=CARTESIAN_POINT('Ctrl Pts',(-12.3296022375865,0.924,40.7164504695946));
#99091=CARTESIAN_POINT('Ctrl Pts',(-11.6999497096383,0.924,39.6710971369163));
#99092=CARTESIAN_POINT('Ctrl Pts',(-11.1874609600943,0.924,38.6392410506538));
#99093=CARTESIAN_POINT('Ctrl Pts',(-11.0113749925991,0.924,37.5398403917748));
#99094=CARTESIAN_POINT('Ctrl Pts',(-11.2537874910971,0.924,36.4518523554272));
#99095=CARTESIAN_POINT('Ctrl Pts',(-11.9032876540853,0.924,35.5613424749907));
#99096=CARTESIAN_POINT('Ctrl Pts',(-12.6910734237184,0.924,35.0111461040952));
#99097=CARTESIAN_POINT('Ctrl Pts',(-13.3725424358171,0.924,34.5834843095939));
#99098=CARTESIAN_POINT('Ctrl Pts',(-13.8907462265714,0.924,34.2368869147185));
#99099=CARTESIAN_POINT('Ctrl Pts',(-14.3877781203166,0.924,33.8201146754649));
#99100=CARTESIAN_POINT('Ctrl Pts',(-14.8238908844334,0.923999999999999,
33.2948194019013));
#99101=CARTESIAN_POINT('Ctrl Pts',(-15.0761879359655,0.924,32.5848794176223));
#99102=CARTESIAN_POINT('Ctrl Pts',(-15.0048415747375,0.924,31.8645500407944));
#99103=CARTESIAN_POINT('Ctrl Pts',(-14.7969073569086,0.924,31.255443467967));
#99104=CARTESIAN_POINT('Ctrl Pts',(-14.4608280370914,0.924,30.4864933436934));
#99105=CARTESIAN_POINT('Ctrl Pts',(-13.8892654107988,0.924,29.1794300100813));
#99106=CARTESIAN_POINT('Ctrl Pts',(-13.3134204366261,0.924,27.3367371289618));
#99107=CARTESIAN_POINT('Ctrl Pts',(-12.676785825845,0.924,25.0072588185284));
#99108=CARTESIAN_POINT('Ctrl Pts',(-12.0379540421531,0.924,22.6694941250056));
#99109=CARTESIAN_POINT('Ctrl Pts',(-11.0930194846002,0.924000000000001,
19.5704317186628));
#99110=CARTESIAN_POINT('Ctrl Pts',(-10.0793574851517,0.924,16.5387499289064));
#99111=CARTESIAN_POINT('Ctrl Pts',(-9.09212599991816,0.924,13.4722442013831));
#99112=CARTESIAN_POINT('Ctrl Pts',(-8.54361306627396,0.924,11.9392205016032));
#99113=CARTESIAN_POINT('Ctrl Pts',(-8.26785692826842,0.924,11.1826993255826));
#99114=CARTESIAN_POINT('Origin',(-7.98599766308436,0.924,11.2854385811275));
#99115=CARTESIAN_POINT('Ctrl Pts',(-7.97548942359086,1.15565058469624,10.3765642386027));
#99116=CARTESIAN_POINT('Ctrl Pts',(-8.06230799714572,1.0034429248949,10.6189650635473));
#99117=CARTESIAN_POINT('Ctrl Pts',(-8.16503623275751,0.92400000000006,10.9006166345145));
#99118=CARTESIAN_POINT('Ctrl Pts',(-8.2678569282683,0.924,11.1826993255823));
#99119=CARTESIAN_POINT('Ctrl Pts',(-7.99045555921432,1.23108469744854,10.4183502697803));
#99120=CARTESIAN_POINT('Ctrl Pts',(-8.07217904790317,1.08475451411851,10.6463513703776));
#99121=CARTESIAN_POINT('Ctrl Pts',(-8.16981771984119,1.00573927772529,10.9134327420293));
#99122=CARTESIAN_POINT('Ctrl Pts',(-8.2678569282683,1.00253981633975,11.1826993255823));
#99123=CARTESIAN_POINT('Ctrl Pts',(-7.94326110749956,1.38102048348872,10.5289633581403));
#99124=CARTESIAN_POINT('Ctrl Pts',(-8.02040943412811,1.24654612868385,10.7271275165187));
#99125=CARTESIAN_POINT('Ctrl Pts',(-8.11273806656634,1.16832799177458,10.9631249146767));
#99126=CARTESIAN_POINT('Ctrl Pts',(-8.20680380061954,1.15901743402805,11.2049535270869));
#99127=CARTESIAN_POINT('Ctrl Pts',(-7.77680414049113,1.42353079316072,10.6151507309428));
#99128=CARTESIAN_POINT('Ctrl Pts',(-7.86054014004693,1.29840666751811,10.8060533124044));
#99129=CARTESIAN_POINT('Ctrl Pts',(-7.95999863022133,1.2290893043484,11.0310584243187));
#99130=CARTESIAN_POINT('Ctrl Pts',(-8.05978824615495,1.22400000000001,11.2585415069226));
#99131=CARTESIAN_POINT('Ctrl Pts',(-7.69305806525894,1.41005007589777,10.6367198785636));
#99132=CARTESIAN_POINT('Ctrl Pts',(-7.78028187341949,1.28780455385259,10.8323127138358));
#99133=CARTESIAN_POINT('Ctrl Pts',(-7.88321097351839,1.22400000000005,11.0589589073799));
#99134=CARTESIAN_POINT('Ctrl Pts',(-7.98599766308424,1.224,11.2854385811272));
#99135=CARTESIAN_POINT('',(-7.69305806525894,1.41005007589777,10.6367198785636));
#99136=CARTESIAN_POINT('Ctrl Pts',(-7.98599766308424,1.224,11.2854385811272));
#99137=CARTESIAN_POINT('Ctrl Pts',(-7.88321097351839,1.22400000000005,11.0589589073799));
#99138=CARTESIAN_POINT('Ctrl Pts',(-7.78028187341949,1.28780455385259,10.8323127138358));
#99139=CARTESIAN_POINT('Ctrl Pts',(-7.69305806525894,1.41005007589777,10.6367198785636));
#99140=CARTESIAN_POINT('Origin',(-7.69305806525894,1.15565058469624,10.4777201965626));
#99141=CARTESIAN_POINT('Ctrl Pts',(-7.69402636887568,1.40836049654452,10.6394232055288));
#99142=CARTESIAN_POINT('Ctrl Pts',(-7.37878397297215,1.9583789756659,9.75939363893455));
#99143=CARTESIAN_POINT('Ctrl Pts',(-7.08515088258527,2.51315943171085,8.87174490926262));
#99144=CARTESIAN_POINT('Ctrl Pts',(-6.90139152215332,3.07969017441782,7.96529572093148));
#99145=CARTESIAN_POINT('Ctrl Pts',(-7.77777254631837,1.42184316271539,10.6178510368671));
#99146=CARTESIAN_POINT('Ctrl Pts',(-7.4624969034848,1.97122882668992,9.7388021111409));
#99147=CARTESIAN_POINT('Ctrl Pts',(-7.16880498204814,2.52378465263871,8.85489320618927));
#99148=CARTESIAN_POINT('Ctrl Pts',(-6.98399462243714,3.08721662507797,7.95325294287824));
#99149=CARTESIAN_POINT('Ctrl Pts',(-7.94428975230827,1.37932471088278,10.5316287085264));
#99150=CARTESIAN_POINT('Ctrl Pts',(-7.6289893652189,1.92813146670491,9.65491827136533));
#99151=CARTESIAN_POINT('Ctrl Pts',(-7.33511759437778,2.4782573725025,8.7798016390015));
#99152=CARTESIAN_POINT('Ctrl Pts',(-7.14841699910981,3.03896615778005,7.88976143408875));
#99153=CARTESIAN_POINT('Ctrl Pts',(-7.99145271748562,1.22929648674672,10.4209666875345));
#99154=CARTESIAN_POINT('Ctrl Pts',(-7.67704649076099,1.77889550193203,9.5452221915896));
#99155=CARTESIAN_POINT('Ctrl Pts',(-7.38682021808006,2.3321450604213,8.67350113810941));
#99156=CARTESIAN_POINT('Ctrl Pts',(-7.2041455986097,2.89666826892147,7.78952721320216));
#99157=CARTESIAN_POINT('Ctrl Pts',(-7.97642326903403,1.15381020723204,10.3791715289931));
#99158=CARTESIAN_POINT('Ctrl Pts',(-7.6626379783708,1.70382952596046,9.50320731474293));
#99159=CARTESIAN_POINT('Ctrl Pts',(-7.3746278026873,2.258613046434,8.63077157801953));
#99160=CARTESIAN_POINT('Ctrl Pts',(-7.19539240778044,2.82514780747502,7.74660133539471));
#99161=CARTESIAN_POINT('',(-6.90195634553822,3.07794992410223,7.96808012143643));
#99162=CARTESIAN_POINT('Origin',(-6.90195634553822,2.8235504329007,7.80908043943548));
#99163=CARTESIAN_POINT('Ctrl Pts',(-7.69305806525894,1.41005007589777,10.6367198785636));
#99164=CARTESIAN_POINT('Ctrl Pts',(-7.37850550563988,1.95895191811054,9.75847693102314));
#99165=CARTESIAN_POINT('Ctrl Pts',(-7.08556384332816,2.512603379587,8.87263459266079));
#99166=CARTESIAN_POINT('Ctrl Pts',(-6.90195634553822,3.07794992410223,7.96808012143643));
#99167=CARTESIAN_POINT('Ctrl Pts',(-7.10945460790939,2.964,7.27219995625739));
#99168=CARTESIAN_POINT('Ctrl Pts',(-7.13617164034088,2.964,7.44003720108978));
#99169=CARTESIAN_POINT('Ctrl Pts',(-7.16707514154032,2.91473210657155,7.60709602897267));
#99170=CARTESIAN_POINT('Ctrl Pts',(-7.19596078944639,2.8235504329007,7.74940308223659));
#99171=CARTESIAN_POINT('Ctrl Pts',(-7.10945460790939,3.04253981633974,7.27219995625739));
#99172=CARTESIAN_POINT('Ctrl Pts',(-7.13849656639519,3.04402078814626,7.45433830770972));
#99173=CARTESIAN_POINT('Ctrl Pts',(-7.17237393335723,2.99262131539692,7.63626955159092));
#99174=CARTESIAN_POINT('Ctrl Pts',(-7.20466995675359,2.89502896886372,7.79230937050473));
#99175=CARTESIAN_POINT('Ctrl Pts',(-7.04529077570142,3.19902831055547,7.28241382259999));
#99176=CARTESIAN_POINT('Ctrl Pts',(-7.07642208754616,3.20333799642574,7.49435291163428));
#99177=CARTESIAN_POINT('Ctrl Pts',(-7.11349156987445,3.14769091692951,7.70773779464215));
#99178=CARTESIAN_POINT('Ctrl Pts',(-7.14894649883125,3.03726886686138,7.89252011776886));
#99179=CARTESIAN_POINT('Ctrl Pts',(-6.89074805761638,3.264,7.30701457683218));
#99180=CARTESIAN_POINT('Ctrl Pts',(-6.91946353963399,3.26635574534166,7.53407746642906));
#99181=CARTESIAN_POINT('Ctrl Pts',(-6.95292678377081,3.20426081663271,7.76083290171336));
#99182=CARTESIAN_POINT('Ctrl Pts',(-6.98456267119525,3.08548589091379,7.95602257453795));
#99183=CARTESIAN_POINT('Ctrl Pts',(-6.8131848044464,3.264,7.31936141887254));
#99184=CARTESIAN_POINT('Ctrl Pts',(-6.8406282557194,3.264,7.5477362807522));
#99185=CARTESIAN_POINT('Ctrl Pts',(-6.87234328942337,3.19873603727695,7.77482234035689));
#99186=CARTESIAN_POINT('Ctrl Pts',(-6.90195634553822,3.07794992410224,7.96808012143643));
#99187=CARTESIAN_POINT('',(-6.8131848044464,3.264,7.31936141887254));
#99188=CARTESIAN_POINT('Ctrl Pts',(-6.90195634553822,3.07794992410224,7.96808012143643));
#99189=CARTESIAN_POINT('Ctrl Pts',(-6.87234328942337,3.19873603727695,7.77482234035689));
#99190=CARTESIAN_POINT('Ctrl Pts',(-6.8406282557194,3.264,7.5477362807522));
#99191=CARTESIAN_POINT('Ctrl Pts',(-6.8131848044464,3.264,7.31936141887254));
#99192=CARTESIAN_POINT('Origin',(-6.8131848044464,2.964,7.31936141887254));
#99193=CARTESIAN_POINT('Ctrl Pts',(-6.8131848044464,3.264,7.31936141887255));
#99194=CARTESIAN_POINT('Ctrl Pts',(-6.77276542502368,3.264,7.06544559579084));
#99195=CARTESIAN_POINT('Ctrl Pts',(-6.74100318491171,3.26399999999999,6.81013961060119));
#99196=CARTESIAN_POINT('Ctrl Pts',(-6.71835209239445,3.264,6.5496683313293));
#99197=CARTESIAN_POINT('Ctrl Pts',(-6.71797603803041,3.264,6.54534447147308));
#99198=CARTESIAN_POINT('Ctrl Pts',(-6.71760000000007,3.264,6.54102059420173));
#99199=CARTESIAN_POINT('Ctrl Pts',(-6.89074805761638,3.264,7.30701457683219));
#99200=CARTESIAN_POINT('Ctrl Pts',(-6.85060859506975,3.264,7.05485515618756));
#99201=CARTESIAN_POINT('Ctrl Pts',(-6.81908071837931,3.26399999999999,6.80141438915615));
#99202=CARTESIAN_POINT('Ctrl Pts',(-6.79659880028861,3.264,6.54288927009049));
#99203=CARTESIAN_POINT('Ctrl Pts',(-6.79621901877148,3.264,6.53852248974404));
#99204=CARTESIAN_POINT('Ctrl Pts',(-6.7958444767614,3.264,6.53421584534326));
#99205=CARTESIAN_POINT('Ctrl Pts',(-7.04528673824326,3.1989628628934,7.28241446529942));
#99206=CARTESIAN_POINT('Ctrl Pts',(-7.00570552018148,3.1989628628934,7.03376395992905));
#99207=CARTESIAN_POINT('Ctrl Pts',(-6.97504274772807,3.19896286289339,6.78861582425716));
#99208=CARTESIAN_POINT('Ctrl Pts',(-6.95249369350636,3.19896286289341,6.52931900008258));
#99209=CARTESIAN_POINT('Ctrl Pts',(-6.95211645163852,3.1989628628934,6.52498147096217));
#99210=CARTESIAN_POINT('Ctrl Pts',(-6.95174044180733,3.1989628628934,6.52065791852088));
#99211=CARTESIAN_POINT('Ctrl Pts',(-7.10945460790939,3.04253981633974,7.27219995625739));
#99212=CARTESIAN_POINT('Ctrl Pts',(-7.07010511574258,3.04253981633974,7.0250051988394));
#99213=CARTESIAN_POINT('Ctrl Pts',(-7.0397495283659,3.04253981633974,6.78270237401318));
#99214=CARTESIAN_POINT('Ctrl Pts',(-7.01722541347195,3.04253981633974,6.52369262500357));
#99215=CARTESIAN_POINT('Ctrl Pts',(-7.01684792393932,3.04253981633974,6.5193522454573));
#99216=CARTESIAN_POINT('Ctrl Pts',(-7.01647188590898,3.04253981633974,6.51502836818595));
#99217=CARTESIAN_POINT('Ctrl Pts',(-7.10945460790939,2.964,7.27219995625739));
#99218=CARTESIAN_POINT('Ctrl Pts',(-7.07010511574258,2.964,7.0250051988394));
#99219=CARTESIAN_POINT('Ctrl Pts',(-7.0397495283659,2.96399999999999,6.78270237401318));
#99220=CARTESIAN_POINT('Ctrl Pts',(-7.01722541347195,2.964,6.52369262500357));
#99221=CARTESIAN_POINT('Ctrl Pts',(-7.01684792393932,2.964,6.5193522454573));
#99222=CARTESIAN_POINT('Ctrl Pts',(-7.01647188590898,2.964,6.51502836818595));
#99223=CARTESIAN_POINT('',(-6.7176,3.264,6.54102059420174));
#99224=CARTESIAN_POINT('Ctrl Pts',(-6.8131848044464,3.264,7.31936141887255));
#99225=CARTESIAN_POINT('Ctrl Pts',(-6.77276542502368,3.264,7.06544559579084));
#99226=CARTESIAN_POINT('Ctrl Pts',(-6.74100318491171,3.26399999999999,6.81013961060119));
#99227=CARTESIAN_POINT('Ctrl Pts',(-6.71835209239445,3.264,6.5496683313293));
#99228=CARTESIAN_POINT('Ctrl Pts',(-6.71797603803041,3.264,6.54534447147308));
#99229=CARTESIAN_POINT('Ctrl Pts',(-6.71760000000007,3.264,6.54102059420173));
#99230=CARTESIAN_POINT('Ctrl Pts',(-6.7176000000002,3.264,6.54102059420098));
#99231=CARTESIAN_POINT('Ctrl Pts',(-6.71833165319913,3.264,6.54120934340536));
#99232=CARTESIAN_POINT('Ctrl Pts',(-6.71906410849758,3.26399732346502,6.54139488274335));
#99233=CARTESIAN_POINT('Ctrl Pts',(-6.74443279705516,3.26381150391108,6.54770283617451));
#99234=CARTESIAN_POINT('Ctrl Pts',(-6.76899387896665,3.26065160540924,6.54990773601873));
#99235=CARTESIAN_POINT('Ctrl Pts',(-6.81740983957415,3.24798417582051,6.54861388368172));
#99236=CARTESIAN_POINT('Ctrl Pts',(-6.84022091954467,3.23887327016054,6.54532375830639));
#99237=CARTESIAN_POINT('Ctrl Pts',(-6.88647361235057,3.21357659218827,6.53744289499075));
#99238=CARTESIAN_POINT('Ctrl Pts',(-6.90943210370148,3.19642495146849,6.53274268516599));
#99239=CARTESIAN_POINT('Ctrl Pts',(-6.94706293362363,3.15880713459934,6.53103362429698));
#99240=CARTESIAN_POINT('Ctrl Pts',(-6.96534422261705,3.13628933865456,6.53291537653795));
#99241=CARTESIAN_POINT('Ctrl Pts',(-6.99299814551648,3.08561018365874,6.53348362099248));
#99242=CARTESIAN_POINT('Ctrl Pts',(-7.00213172179733,3.06230910196935,6.53267399033088));
#99243=CARTESIAN_POINT('Ctrl Pts',(-7.0147942159154,3.01264906168983,6.52984196355258));
#99244=CARTESIAN_POINT('Ctrl Pts',(-7.0176,2.98769953894126,6.52800007780761));
#99245=CARTESIAN_POINT('Ctrl Pts',(-7.0176,2.964,6.52800007780761));
#99246=CARTESIAN_POINT('Origin',(-6.7176,2.964,-19.584));
#99247=CARTESIAN_POINT('',(-6.7176,3.264,-14.688));
#99248=CARTESIAN_POINT('',(-6.7176,3.264,-19.584));
#99249=CARTESIAN_POINT('',(-7.0176,2.964,-14.688));
#99250=CARTESIAN_POINT('Origin',(-6.7176,2.964,-14.688));
#99251=CARTESIAN_POINT('',(-7.0176,2.964,-19.584));
#99252=CARTESIAN_POINT('Origin',(0.,2.964,-14.688));
#99253=CARTESIAN_POINT('',(6.7176,3.264,-14.688));
#99254=CARTESIAN_POINT('',(7.0176,2.964,-14.688));
#99255=CARTESIAN_POINT('Origin',(6.7176,2.964,-14.688));
#99256=CARTESIAN_POINT('Origin',(0.,2.964,-14.688));
#99257=CARTESIAN_POINT('Origin',(0.,3.264,-14.688));
#99258=CARTESIAN_POINT('Origin',(6.7176,2.964,-8.976));
#99259=CARTESIAN_POINT('',(7.0176,2.964,-8.976));
#99260=CARTESIAN_POINT('',(6.71760000000007,3.264,6.54102059420079));
#99261=CARTESIAN_POINT('',(6.7176,3.264,-8.976));
#99262=CARTESIAN_POINT('Ctrl Pts',(6.71760000000026,3.264,6.54102059420005));
#99263=CARTESIAN_POINT('Ctrl Pts',(6.71833161535042,3.264,6.54121031917896));
#99264=CARTESIAN_POINT('Ctrl Pts',(6.71906402903224,3.26399732374162,6.54139686702817));
#99265=CARTESIAN_POINT('Ctrl Pts',(6.744304090703,3.26381245686305,6.54770905827349));
#99266=CARTESIAN_POINT('Ctrl Pts',(6.76874616727742,3.26068433500669,6.54999627440179));
#99267=CARTESIAN_POINT('Ctrl Pts',(6.81694811446642,3.24813572935757,6.54892168893177));
#99268=CARTESIAN_POINT('Ctrl Pts',(6.83966741557286,3.23911015473846,6.54576286024958));
#99269=CARTESIAN_POINT('Ctrl Pts',(6.88609886105684,3.21385739564275,6.53802232312692));
#99270=CARTESIAN_POINT('Ctrl Pts',(6.90926565630398,3.1965906610116,6.53330291862062));
#99271=CARTESIAN_POINT('Ctrl Pts',(6.94715428211924,3.15871639917427,6.53154772477979));
#99272=CARTESIAN_POINT('Ctrl Pts',(6.96558458258161,3.13600641445292,6.53338605654475));
#99273=CARTESIAN_POINT('Ctrl Pts',(6.99322546109818,3.08507067475937,6.53373480681712));
#99274=CARTESIAN_POINT('Ctrl Pts',(7.00227690287596,3.06185555957858,6.53282707247597));
#99275=CARTESIAN_POINT('Ctrl Pts',(7.01481452566474,3.01244578554285,6.52986850096268));
#99276=CARTESIAN_POINT('Ctrl Pts',(7.0176,2.98761215526521,6.528000078773));
#99277=CARTESIAN_POINT('Ctrl Pts',(7.0176,2.964,6.528000078773));
#99278=CARTESIAN_POINT('Ctrl Pts',(7.1959607894463,2.8235504329007,7.74940308223601));
#99279=CARTESIAN_POINT('Ctrl Pts',(7.16707443778447,2.91473432807616,7.60709256187426));
#99280=CARTESIAN_POINT('Ctrl Pts',(7.13617229126044,2.964,7.44004129019165));
#99281=CARTESIAN_POINT('Ctrl Pts',(7.10945460790829,2.964,7.27219995625688));
#99282=CARTESIAN_POINT('Ctrl Pts',(7.20466995675359,2.89502896886377,7.79230937050415));
#99283=CARTESIAN_POINT('Ctrl Pts',(7.1723731465128,2.99262369308791,7.63626574991444));
#99284=CARTESIAN_POINT('Ctrl Pts',(7.13849727395811,3.04402082422793,7.45434274523658));
#99285=CARTESIAN_POINT('Ctrl Pts',(7.10945460790829,3.04253981633974,7.27219995625688));
#99286=CARTESIAN_POINT('Ctrl Pts',(7.14894649883135,3.03726886686152,7.89252011776843));
#99287=CARTESIAN_POINT('Ctrl Pts',(7.11349070606817,3.14769360719685,7.70773329269815));
#99288=CARTESIAN_POINT('Ctrl Pts',(7.07642284601308,3.20333810142481,7.49435807521152));
#99289=CARTESIAN_POINT('Ctrl Pts',(7.04529077570034,3.19902831055547,7.2824138225996));
#99290=CARTESIAN_POINT('Ctrl Pts',(6.9845626711953,3.08548589091386,7.95602257453783));
#99291=CARTESIAN_POINT('Ctrl Pts',(6.95292601300975,3.2042637104052,7.76082814621037));
#99292=CARTESIAN_POINT('Ctrl Pts',(6.91946423924288,3.26635580273589,7.53408299847537));
#99293=CARTESIAN_POINT('Ctrl Pts',(6.89074805761534,3.264,7.30701457683205));
#99294=CARTESIAN_POINT('Ctrl Pts',(6.90195634553824,3.07794992410223,7.96808012143643));
#99295=CARTESIAN_POINT('Ctrl Pts',(6.87234256794554,3.19873898004894,7.77481763192169));
#99296=CARTESIAN_POINT('Ctrl Pts',(6.84062892433718,3.264,7.54774184476293));
#99297=CARTESIAN_POINT('Ctrl Pts',(6.81318480444538,3.264,7.31936141887254));
#99298=CARTESIAN_POINT('',(6.81318480444538,3.264,7.31936141887254));
#99299=CARTESIAN_POINT('Origin',(6.81318480444538,2.964,7.31936141887254));
#99300=CARTESIAN_POINT('',(6.90195634553824,3.07794992410223,7.96808012143643));
#99301=CARTESIAN_POINT('Ctrl Pts',(6.81318480444538,3.264,7.31936141887254));
#99302=CARTESIAN_POINT('Ctrl Pts',(6.84062892433718,3.264,7.54774184476293));
#99303=CARTESIAN_POINT('Ctrl Pts',(6.87234256794554,3.19873898004894,7.77481763192169));
#99304=CARTESIAN_POINT('Ctrl Pts',(6.90195634553824,3.07794992410223,7.96808012143643));
#99305=CARTESIAN_POINT('Origin',(6.90195634553824,2.8235504329007,7.80908043943548));
#99306=CARTESIAN_POINT('Ctrl Pts',(6.71760000000007,3.264,6.54102059420079));
#99307=CARTESIAN_POINT('Ctrl Pts',(6.71797603803036,3.264,6.54534447147182));
#99308=CARTESIAN_POINT('Ctrl Pts',(6.71835209239434,3.264,6.54966833132773));
#99309=CARTESIAN_POINT('Ctrl Pts',(6.74100318491002,3.264,6.81013961059996));
#99310=CARTESIAN_POINT('Ctrl Pts',(6.77276542502211,3.264,7.0654455957901));
#99311=CARTESIAN_POINT('Ctrl Pts',(6.81318480444533,3.264,7.31936141887222));
#99312=CARTESIAN_POINT('Ctrl Pts',(6.79584447676144,3.264,6.53421584534281));
#99313=CARTESIAN_POINT('Ctrl Pts',(6.79621901877147,3.264,6.53852248974327));
#99314=CARTESIAN_POINT('Ctrl Pts',(6.79659880028854,3.264,6.54288927008942));
#99315=CARTESIAN_POINT('Ctrl Pts',(6.81908071837765,3.264,6.80141438915507));
#99316=CARTESIAN_POINT('Ctrl Pts',(6.85060859506817,3.264,7.05485515618676));
#99317=CARTESIAN_POINT('Ctrl Pts',(6.89074805761529,3.264,7.30701457683173));
#99318=CARTESIAN_POINT('Ctrl Pts',(6.95166378082186,3.19894727191536,6.52066458555755));
#99319=CARTESIAN_POINT('Ctrl Pts',(6.95203954305117,3.19894727191536,6.52498528583783));
#99320=CARTESIAN_POINT('Ctrl Pts',(6.9524209881539,3.19894727191536,6.52937115569764));
#99321=CARTESIAN_POINT('Ctrl Pts',(6.97463672769311,3.19894727191537,6.78483527185625));
#99322=CARTESIAN_POINT('Ctrl Pts',(7.00562922258625,3.19894727191536,7.03377380853805));
#99323=CARTESIAN_POINT('Ctrl Pts',(7.0452107446937,3.19894727191536,7.2824265622686));
#99324=CARTESIAN_POINT('Ctrl Pts',(7.01647188590914,3.04253981633974,6.51502836818689));
#99325=CARTESIAN_POINT('Ctrl Pts',(7.01684792393943,3.04253981633974,6.51935224545793));
#99326=CARTESIAN_POINT('Ctrl Pts',(7.0172303787086,3.04253981633974,6.52374971782953));
#99327=CARTESIAN_POINT('Ctrl Pts',(7.03933150750459,3.04253981633974,6.77789575673342));
#99328=CARTESIAN_POINT('Ctrl Pts',(7.07010511574098,3.04253981633974,7.02500519883843));
#99329=CARTESIAN_POINT('Ctrl Pts',(7.10945460790824,3.04253981633974,7.27219995625657));
#99330=CARTESIAN_POINT('Ctrl Pts',(7.01647188590914,2.964,6.51502836818689));
#99331=CARTESIAN_POINT('Ctrl Pts',(7.01684792393943,2.964,6.51935224545793));
#99332=CARTESIAN_POINT('Ctrl Pts',(7.0172303787086,2.964,6.52374971782953));
#99333=CARTESIAN_POINT('Ctrl Pts',(7.03933150750459,2.964,6.77789575673342));
#99334=CARTESIAN_POINT('Ctrl Pts',(7.07010511574098,2.964,7.02500519883843));
#99335=CARTESIAN_POINT('Ctrl Pts',(7.10945460790824,2.964,7.27219995625657));
#99336=CARTESIAN_POINT('Ctrl Pts',(6.71760000000007,3.264,6.54102059420079));
#99337=CARTESIAN_POINT('Ctrl Pts',(6.71797603803036,3.264,6.54534447147182));
#99338=CARTESIAN_POINT('Ctrl Pts',(6.71835209239434,3.264,6.54966833132773));
#99339=CARTESIAN_POINT('Ctrl Pts',(6.74100318491002,3.264,6.81013961059996));
#99340=CARTESIAN_POINT('Ctrl Pts',(6.77276542502211,3.264,7.0654455957901));
#99341=CARTESIAN_POINT('Ctrl Pts',(6.81318480444533,3.264,7.31936141887222));
#99342=CARTESIAN_POINT('Ctrl Pts',(6.90139152214811,3.07969017443392,7.96529572090572));
#99343=CARTESIAN_POINT('Ctrl Pts',(7.08515088258326,2.51315943171628,8.87174490925396));
#99344=CARTESIAN_POINT('Ctrl Pts',(7.37878397297277,1.95837897566052,9.75939363894316));
#99345=CARTESIAN_POINT('Ctrl Pts',(7.69402636888245,1.40836049652889,10.6394232055538));
#99346=CARTESIAN_POINT('Ctrl Pts',(6.98399462243194,3.08721662509406,7.9532529428525));
#99347=CARTESIAN_POINT('Ctrl Pts',(7.16880498204613,2.52378465264413,8.85489320618061));
#99348=CARTESIAN_POINT('Ctrl Pts',(7.46249690348542,1.97122882668447,9.7388021111496));
#99349=CARTESIAN_POINT('Ctrl Pts',(7.77777254632515,1.42184316269977,10.6178510368922));
#99350=CARTESIAN_POINT('Ctrl Pts',(7.14841699910512,3.03896615779599,7.88976143406284));
#99351=CARTESIAN_POINT('Ctrl Pts',(7.33511759437628,2.47825737250777,8.77980163899264));
#99352=CARTESIAN_POINT('Ctrl Pts',(7.62898936522003,1.92813146669928,9.654918271374));
#99353=CARTESIAN_POINT('Ctrl Pts',(7.94428975231557,1.37932471086703,10.531628708551));
#99354=CARTESIAN_POINT('Ctrl Pts',(7.20414559860485,2.89666826893669,7.78952721317584));
#99355=CARTESIAN_POINT('Ctrl Pts',(7.38682021807838,2.33214506042582,8.67350113810013));
#99356=CARTESIAN_POINT('Ctrl Pts',(7.67704649076199,1.7788955019257,9.54522219159796));
#99357=CARTESIAN_POINT('Ctrl Pts',(7.99145271749268,1.22929648673017,10.4209666875588));
#99358=CARTESIAN_POINT('Ctrl Pts',(7.19539240777509,2.8251478074898,7.74660133536821));
#99359=CARTESIAN_POINT('Ctrl Pts',(7.37462780268508,2.25861304643806,8.6307715780101));
#99360=CARTESIAN_POINT('Ctrl Pts',(7.6626379783713,1.70382952595369,9.50320731475117));
#99361=CARTESIAN_POINT('Ctrl Pts',(7.9764232690405,1.153810207215,10.3791715290174));
#99362=CARTESIAN_POINT('',(7.69305806525675,1.41005007589777,10.6367198785636));
#99363=CARTESIAN_POINT('Origin',(7.69305806525675,1.15565058469624,10.4777201965626));
#99364=CARTESIAN_POINT('Ctrl Pts',(6.90195634553824,3.07794992410223,7.96808012143643));
#99365=CARTESIAN_POINT('Ctrl Pts',(7.08556384332996,2.51260337958728,8.87263459266035));
#99366=CARTESIAN_POINT('Ctrl Pts',(7.37850550563793,1.95895191811046,9.75847693102326));
#99367=CARTESIAN_POINT('Ctrl Pts',(7.69305806525675,1.41005007589777,10.6367198785636));
#99368=CARTESIAN_POINT('Ctrl Pts',(8.26785692826664,0.924,11.1826993255823));
#99369=CARTESIAN_POINT('Ctrl Pts',(8.16503869361036,0.924000000000001,10.900623385729));
#99370=CARTESIAN_POINT('Ctrl Pts',(8.06230591927477,1.00344656775053,10.6189592620572));
#99371=CARTESIAN_POINT('Ctrl Pts',(7.97548942358868,1.15565058469624,10.3765642386028));
#99372=CARTESIAN_POINT('Ctrl Pts',(8.26785692826664,1.00253981633975,11.1826993255823));
#99373=CARTESIAN_POINT('Ctrl Pts',(8.16982006625653,1.00573920115106,10.9134391865099));
#99374=CARTESIAN_POINT('Ctrl Pts',(8.07217709197523,1.08475801630582,10.6463459135227));
#99375=CARTESIAN_POINT('Ctrl Pts',(7.99045555921214,1.23108469744854,10.4183502697804));
#99376=CARTESIAN_POINT('Ctrl Pts',(8.20680380061789,1.15901743402804,11.2049535270869));
#99377=CARTESIAN_POINT('Ctrl Pts',(8.11274031788272,1.1683277689407,10.9631307024719));
#99378=CARTESIAN_POINT('Ctrl Pts',(8.02040758769964,1.2465493471202,10.7271227737651));
#99379=CARTESIAN_POINT('Ctrl Pts',(7.94326110749736,1.38102048348871,10.5289633581403));
#99380=CARTESIAN_POINT('Ctrl Pts',(8.05978824615337,1.224,11.2585415069228));
#99381=CARTESIAN_POINT('Ctrl Pts',(7.96000101853004,1.22908918254371,11.0310638687758));
#99382=CARTESIAN_POINT('Ctrl Pts',(7.86053813595267,1.29840966217113,10.8060487434454));
#99383=CARTESIAN_POINT('Ctrl Pts',(7.77680414048894,1.42353079316071,10.6151507309429));
#99384=CARTESIAN_POINT('Ctrl Pts',(7.98599766308269,1.224,11.2854385811275));
#99385=CARTESIAN_POINT('Ctrl Pts',(7.88321343355745,1.224,11.0589643278221));
#99386=CARTESIAN_POINT('Ctrl Pts',(7.7802797858499,1.28780747961066,10.8323080326229));
#99387=CARTESIAN_POINT('Ctrl Pts',(7.69305806525675,1.41005007589777,10.6367198785636));
#99388=CARTESIAN_POINT('Ctrl Pts',(7.69305806525675,1.41005007589777,10.6367198785636));
#99389=CARTESIAN_POINT('Ctrl Pts',(7.7802797858499,1.28780747961066,10.8323080326229));
#99390=CARTESIAN_POINT('Ctrl Pts',(7.88321343355745,1.224,11.0589643278221));
#99391=CARTESIAN_POINT('Ctrl Pts',(7.98599766308269,1.224,11.2854385811275));
#99392=CARTESIAN_POINT('Origin',(-7.0176,-4.08,-14.688));
#99393=CARTESIAN_POINT('',(-7.0176,2.448,-14.688));
#99394=CARTESIAN_POINT('',(-7.0176,-4.08,-14.688));
#99395=CARTESIAN_POINT('',(-7.0176,2.448,6.99296141887254));
#99396=CARTESIAN_POINT('',(-7.0176,2.448,-3.672));
#99397=CARTESIAN_POINT('',(-7.0176,2.26194992410223,7.64168012143644));
#99398=CARTESIAN_POINT('Origin',(-7.0176,1.224,6.99296141887254));
#99399=CARTESIAN_POINT('',(-7.01760431834114,1.93536901811185,8.16420957102104));
#99400=CARTESIAN_POINT('',(-7.0176,5.46215730337078,2.52134831460674));
#99401=CARTESIAN_POINT('',(-7.01770541278284,2.29368306071046,7.63779914846271));
#99402=CARTESIAN_POINT('Origin',(-7.0176,3.0385827613015,7.37874354812469));
#99403=CARTESIAN_POINT('',(-7.01761410688719,2.58763798856244,6.96055221898186));
#99404=CARTESIAN_POINT('Ctrl Pts',(-7.0176,2.29351434713884,7.63766291347531));
#99405=CARTESIAN_POINT('Ctrl Pts',(-7.0176,2.3740423712826,7.52757570477833));
#99406=CARTESIAN_POINT('Ctrl Pts',(-7.01759999999634,2.44050724085831,7.40695060784198));
#99407=CARTESIAN_POINT('Ctrl Pts',(-7.01759999999634,2.53393775667856,7.17694898676314));
#99408=CARTESIAN_POINT('Ctrl Pts',(-7.0176,2.56551852364822,7.07078797586639));
#99409=CARTESIAN_POINT('Ctrl Pts',(-7.0176,2.58767722915247,6.96056009343683));
#99410=CARTESIAN_POINT('Ctrl Pts',(-7.0176,2.58761674131499,6.96054790557659));
#99411=CARTESIAN_POINT('Ctrl Pts',(-7.0176,2.59970615397228,6.90071766460443));
#99412=CARTESIAN_POINT('Ctrl Pts',(-7.0176,2.61360398776887,6.83777005305424));
#99413=CARTESIAN_POINT('Ctrl Pts',(-7.0176,2.63916505855607,6.73818458534492));
#99414=CARTESIAN_POINT('Ctrl Pts',(-7.01759999998582,2.65165291111849,6.69372255866987));
#99415=CARTESIAN_POINT('Ctrl Pts',(-7.01759999998582,2.68155149694533,6.60703862938188));
#99416=CARTESIAN_POINT('Ctrl Pts',(-7.0176,2.69834666935346,6.56963566225437));
#99417=CARTESIAN_POINT('Ctrl Pts',(-7.0176,2.72097423429567,6.54173976032029));
#99418=CARTESIAN_POINT('Ctrl Pts',(-7.01759999999971,2.7266719134448,6.5361535692381));
#99419=CARTESIAN_POINT('Ctrl Pts',(-7.01759999999971,2.73523606353071,6.53109114103823));
#99420=CARTESIAN_POINT('Ctrl Pts',(-7.0176,2.73773933071856,6.52993454070379));
#99421=CARTESIAN_POINT('Ctrl Pts',(-7.0176,2.74285825285848,6.52839954478026));
#99422=CARTESIAN_POINT('Ctrl Pts',(-7.0176,2.74540196897649,6.52799999999999));
#99423=CARTESIAN_POINT('Ctrl Pts',(-7.0176,2.748,6.52799999999999));
#99424=CARTESIAN_POINT('Origin',(0.,-4.08,-14.688));
#99425=CARTESIAN_POINT('',(7.0176,2.448,-14.688));
#99426=CARTESIAN_POINT('',(7.0176,-4.08,-14.688));
#99427=CARTESIAN_POINT('Origin',(0.,2.448,-14.688));
#99428=CARTESIAN_POINT('Origin',(7.0176,-4.08,6.528));
#99429=CARTESIAN_POINT('',(7.01761391330466,2.5876376799666,6.96055224393119));
#99430=CARTESIAN_POINT('Ctrl Pts',(7.0176,2.748,6.52799999999999));
#99431=CARTESIAN_POINT('Ctrl Pts',(7.0176,2.74511036893714,6.52799999999999));
#99432=CARTESIAN_POINT('Ctrl Pts',(7.0176,2.74229339126459,6.52849427846896));
#99433=CARTESIAN_POINT('Ctrl Pts',(7.0176,2.73662501896236,6.53037541474026));
#99434=CARTESIAN_POINT('Ctrl Pts',(7.0176,2.73386178483929,6.53179413745192));
#99435=CARTESIAN_POINT('Ctrl Pts',(7.0176,2.72454608146371,6.5378716410484));
#99436=CARTESIAN_POINT('Ctrl Pts',(7.0176,2.71812411704449,6.54466757895269));
#99437=CARTESIAN_POINT('Ctrl Pts',(7.0176,2.69356885127018,6.57837479338247));
#99438=CARTESIAN_POINT('Ctrl Pts',(7.01760000001758,2.67322594731515,6.62433548265231));
#99439=CARTESIAN_POINT('Ctrl Pts',(7.01760000001758,2.62579638706691,6.78269963358924));
#99440=CARTESIAN_POINT('Ctrl Pts',(7.0176,2.60429557786619,6.87800461107322));
#99441=CARTESIAN_POINT('Ctrl Pts',(7.0176,2.58761652893502,6.9605489566511));
#99442=CARTESIAN_POINT('',(7.01770541278263,2.2936830607088,7.63779914846461));
#99443=CARTESIAN_POINT('Ctrl Pts',(7.0176,2.58767682077497,6.960562124904));
#99444=CARTESIAN_POINT('Ctrl Pts',(7.0176,2.56298409413704,7.08339472961271));
#99445=CARTESIAN_POINT('Ctrl Pts',(7.01759999990208,2.52660430658189,7.20111310457098));
#99446=CARTESIAN_POINT('Ctrl Pts',(7.01759999990208,2.42819109620806,7.42898400669956));
#99447=CARTESIAN_POINT('Ctrl Pts',(7.0176,2.36665124679277,7.53767986755727));
#99448=CARTESIAN_POINT('Ctrl Pts',(7.0176,2.29351434713977,7.63766291347403));
#99449=CARTESIAN_POINT('',(7.01760411951713,1.93536442690257,8.16421691695589));
#99450=CARTESIAN_POINT('Origin',(7.0176,3.00424770096522,7.39945472980219));
#99451=CARTESIAN_POINT('',(7.0176,2.26194992410223,7.64168012143644));
#99452=CARTESIAN_POINT('',(7.0176,0.694516853932584,10.1495730337079));
#99453=CARTESIAN_POINT('',(7.0176,2.448,6.99296141887254));
#99454=CARTESIAN_POINT('Origin',(7.0176,1.224,6.99296141887254));
#99455=CARTESIAN_POINT('',(7.0176,2.448,6.936));
#99456=CARTESIAN_POINT('Origin',(12.648,-4.08,45.696));
#99457=CARTESIAN_POINT('Ctrl Pts',(7.69004994112325,0.594050075897773,10.3103198785636));
#99458=CARTESIAN_POINT('Ctrl Pts',(7.37565292717766,1.14292103979677,9.43212633632517));
#99459=CARTESIAN_POINT('Ctrl Pts',(7.08320222221595,1.69659760459055,8.54624383265512));
#99460=CARTESIAN_POINT('Ctrl Pts',(6.90025424549142,2.26194992410223,7.64168012143644));
#99461=CARTESIAN_POINT('Ctrl Pts',(7.7566099417083,0.604759632121113,10.2931845886062));
#99462=CARTESIAN_POINT('Ctrl Pts',(7.44282948876134,1.15322808712422,9.41561937075493));
#99463=CARTESIAN_POINT('Ctrl Pts',(7.15265898639664,1.70551531081992,8.53207367891967));
#99464=CARTESIAN_POINT('Ctrl Pts',(6.97247659379773,2.26851485319919,7.6311762348813));
#99465=CARTESIAN_POINT('Ctrl Pts',(7.88938556140221,0.668907343792859,10.2857426732368));
#99466=CARTESIAN_POINT('Ctrl Pts',(7.57681706437755,1.21707193313268,9.40974380083994));
#99467=CARTESIAN_POINT('Ctrl Pts',(7.29124285060054,1.76814635786057,8.53186871114456));
#99468=CARTESIAN_POINT('Ctrl Pts',(7.11645477354901,2.3292995967516,7.64004711813782));
#99469=CARTESIAN_POINT('Ctrl Pts',(7.96060515342953,0.788498764169074,10.3349903948698));
#99470=CARTESIAN_POINT('Ctrl Pts',(7.64807518901572,1.3371289727315,9.46045329326645));
#99471=CARTESIAN_POINT('Ctrl Pts',(7.36254955939489,1.88994777765749,8.58798846944997));
#99472=CARTESIAN_POINT('Ctrl Pts',(7.18671249288602,2.4538649372709,7.70369083485712));
#99473=CARTESIAN_POINT('Ctrl Pts',(7.97249537063514,0.848449567099299,10.3682028984962));
#99474=CARTESIAN_POINT('Ctrl Pts',(7.65957903289365,1.3973205309983,9.49414527429423));
#99475=CARTESIAN_POINT('Ctrl Pts',(7.37274783895485,1.95099709579208,8.62351966308874));
#99476=CARTESIAN_POINT('Ctrl Pts',(7.19430053092001,2.51634941530375,7.74120895321939));
#99477=CARTESIAN_POINT('Origin',(6.90025424549142,2.51634941530375,7.80067980343739));
#99478=CARTESIAN_POINT('',(7.69004994112325,0.594050075897772,10.3103198785636));
#99479=CARTESIAN_POINT('Origin',(7.69004994112325,0.848449567099299,10.4693195605645));
#99480=CARTESIAN_POINT('Ctrl Pts',(7.69004994112325,0.594050075897773,10.3103198785636));
#99481=CARTESIAN_POINT('Ctrl Pts',(7.43642528501577,1.03682530368781,9.6018795140995));
#99482=CARTESIAN_POINT('Ctrl Pts',(7.19708258213954,1.4827278622412,8.88843542041408));
#99483=CARTESIAN_POINT('Ctrl Pts',(7.0179868222806,1.93536441515841,8.16421693574654));
#99484=CARTESIAN_POINT('Ctrl Pts',(7.06362916696882,2.7480230090648,6.95414127896201));
#99485=CARTESIAN_POINT('Ctrl Pts',(7.0993690878108,2.74811551919964,7.23155382342856));
#99486=CARTESIAN_POINT('Ctrl Pts',(7.14696080934769,2.66643382276424,7.5071905074376));
#99487=CARTESIAN_POINT('Ctrl Pts',(7.19438354265699,2.51611178510552,7.74161935745458));
#99488=CARTESIAN_POINT('Ctrl Pts',(7.06363490740171,2.69944028986368,6.95415602179895));
#99489=CARTESIAN_POINT('Ctrl Pts',(7.09821965127004,2.70026704502072,7.22262797399989));
#99490=CARTESIAN_POINT('Ctrl Pts',(7.14400277235035,2.62236748381514,7.49012436326919));
#99491=CARTESIAN_POINT('Ctrl Pts',(7.18969017835144,2.47747072284844,7.7184010716774));
#99492=CARTESIAN_POINT('Ctrl Pts',(7.03586871828684,2.5860173677501,6.95776948019296));
#99493=CARTESIAN_POINT('Ctrl Pts',(7.06872790702351,2.58856514291509,7.20598605294365));
#99494=CARTESIAN_POINT('Ctrl Pts',(7.11175827397579,2.51949133545424,7.45491010747032));
#99495=CARTESIAN_POINT('Ctrl Pts',(7.15489990897123,2.38727021999165,7.66902358769554));
#99496=CARTESIAN_POINT('Ctrl Pts',(6.95031555185498,2.50367339927269,6.96881823558572));
#99497=CARTESIAN_POINT('Ctrl Pts',(6.98392692928157,2.50655355403587,7.20376129641692));
#99498=CARTESIAN_POINT('Ctrl Pts',(7.02813588214951,2.44235324221148,7.4396687902832));
#99499=CARTESIAN_POINT('Ctrl Pts',(7.07234001721698,2.31860209564757,7.64277634582262));
#99500=CARTESIAN_POINT('Ctrl Pts',(6.89212767908006,2.47624041956814,6.97632364997776));
#99501=CARTESIAN_POINT('Ctrl Pts',(6.9266553668271,2.47850902575585,7.20761906768847));
#99502=CARTESIAN_POINT('Ctrl Pts',(6.9721868803631,2.41488748239933,7.43917519062995));
#99503=CARTESIAN_POINT('Ctrl Pts',(7.01767749054815,2.29330136612035,7.63800974414734));
#99504=CARTESIAN_POINT('Origin',(6.76615104985734,2.748,6.99296141887254));
#99505=CARTESIAN_POINT('Ctrl Pts',(7.0176,2.58761550237112,6.96055403711337));
#99506=CARTESIAN_POINT('Ctrl Pts',(6.99922349531616,2.58761550237112,6.81797069470138));
#99507=CARTESIAN_POINT('Ctrl Pts',(6.98374576415963,2.58761550237112,6.67509413737213));
#99508=CARTESIAN_POINT('Ctrl Pts',(6.97130347175975,2.58761550237112,6.53202630652935));
#99509=CARTESIAN_POINT('Ctrl Pts',(7.04750769996015,2.63528330527516,6.95669945649334));
#99510=CARTESIAN_POINT('Ctrl Pts',(7.0291833743663,2.63528330527516,6.81452097176143));
#99511=CARTESIAN_POINT('Ctrl Pts',(7.01375047339114,2.63528330527516,6.6720564108619));
#99512=CARTESIAN_POINT('Ctrl Pts',(7.00134514825194,2.63528330527516,6.52941364845733));
#99513=CARTESIAN_POINT('Ctrl Pts',(7.06369006012584,2.69159478975873,6.95461383265853));
#99514=CARTESIAN_POINT('Ctrl Pts',(7.04539389161563,2.69159478975873,6.81265381880386));
#99515=CARTESIAN_POINT('Ctrl Pts',(7.02998537672209,2.69159478975873,6.67041338531935));
#99516=CARTESIAN_POINT('Ctrl Pts',(7.0176,2.69159478975873,6.52799999999999));
#99517=CARTESIAN_POINT('Ctrl Pts',(7.06369006012584,2.748,6.95461383265853));
#99518=CARTESIAN_POINT('Ctrl Pts',(7.04539374054096,2.748,6.81265264661519));
#99519=CARTESIAN_POINT('Ctrl Pts',(7.02998548375378,2.748,6.67041461602444));
#99520=CARTESIAN_POINT('Ctrl Pts',(7.0176,2.748,6.52799999999999));
#99521=CARTESIAN_POINT('Ctrl Pts',(7.97238210650129,0.848667810146576,10.3678865203214));
#99522=CARTESIAN_POINT('Ctrl Pts',(8.02503872423604,0.756217482327583,10.5149731412681));
#99523=CARTESIAN_POINT('Ctrl Pts',(8.0869221616882,0.707947174569549,10.6858877147699));
#99524=CARTESIAN_POINT('Ctrl Pts',(8.14912361676156,0.708019010352448,10.8568386685929));
#99525=CARTESIAN_POINT('Ctrl Pts',(7.96048761218596,0.788731610271414,10.3346498829601));
#99526=CARTESIAN_POINT('Ctrl Pts',(8.01637706856055,0.687463302222747,10.4908448248288));
#99527=CARTESIAN_POINT('Ctrl Pts',(8.08215444077848,0.632587778955639,10.673073122701));
#99528=CARTESIAN_POINT('Ctrl Pts',(8.14913906922441,0.629465787637592,10.8568651972294));
#99529=CARTESIAN_POINT('Ctrl Pts',(7.88930781714838,0.669130461784413,10.2853123218851));
#99530=CARTESIAN_POINT('Ctrl Pts',(7.94769055067623,0.550421641857097,10.4612353255528));
#99531=CARTESIAN_POINT('Ctrl Pts',(8.01711568751401,0.482182663833425,10.6678349016059));
#99532=CARTESIAN_POINT('Ctrl Pts',(8.08808615036449,0.472961311892119,10.8791433605056));
#99533=CARTESIAN_POINT('Ctrl Pts',(7.75648913737719,0.605033293429871,10.2927630564965));
#99534=CARTESIAN_POINT('Ctrl Pts',(7.81126536355006,0.480889739048768,10.4838995104295));
#99535=CARTESIAN_POINT('Ctrl Pts',(7.87574497017474,0.412984275736593,10.7069427306825));
#99536=CARTESIAN_POINT('Ctrl Pts',(7.94101805558994,0.407988882551097,10.9326817955771));
#99537=CARTESIAN_POINT('Ctrl Pts',(7.68993326017409,0.594320041958723,10.3098881354259));
#99538=CARTESIAN_POINT('Ctrl Pts',(7.74283997308695,0.471850558728837,10.5056555873966));
#99539=CARTESIAN_POINT('Ctrl Pts',(7.80491620373074,0.407905964356365,10.7327647510929));
#99540=CARTESIAN_POINT('Ctrl Pts',(7.86720541257493,0.408000103793674,10.9595386471955));
#99541=CARTESIAN_POINT('Ctrl Pts',(7.86706805722616,0.408,10.9590385811275));
#99542=CARTESIAN_POINT('Ctrl Pts',(7.80487073631488,0.408,10.7325975869917));
#99543=CARTESIAN_POINT('Ctrl Pts',(7.74289233196934,0.471846546370078,10.5058455258079));
#99544=CARTESIAN_POINT('Ctrl Pts',(7.69004994112325,0.594050075897772,10.3103198785636));
#99545=CARTESIAN_POINT('Origin',(0.,1.632,10.9590385811275));
#99546=CARTESIAN_POINT('',(-7.69004994112544,0.594050075897772,10.3103198785636));
#99547=CARTESIAN_POINT('Ctrl Pts',(-7.69004994112544,0.594050075897771,
10.3103198785636));
#99548=CARTESIAN_POINT('Ctrl Pts',(-7.74289233197148,0.471846546370226,
10.5058455258076));
#99549=CARTESIAN_POINT('Ctrl Pts',(-7.80487073631704,0.407999999999999,
10.7325975869917));
#99550=CARTESIAN_POINT('Ctrl Pts',(-7.86706805722818,0.408,10.9590385811275));
#99551=CARTESIAN_POINT('',(0.,0.594050075897772,10.3103198785636));
#99552=CARTESIAN_POINT('Ctrl Pts',(-6.90025424549141,2.26194992410223,7.64168012143643));
#99553=CARTESIAN_POINT('Ctrl Pts',(-7.08320222221414,1.69659760459028,8.54624383265556));
#99554=CARTESIAN_POINT('Ctrl Pts',(-7.37565292717963,1.14292103979685,9.43212633632503));
#99555=CARTESIAN_POINT('Ctrl Pts',(-7.69004994112544,0.594050075897773,
10.3103198785636));
#99556=CARTESIAN_POINT('Ctrl Pts',(-6.97247659379779,2.26851485319913,7.63117623488139));
#99557=CARTESIAN_POINT('Ctrl Pts',(-7.15265898639484,1.70551531081965,8.5320736789201));
#99558=CARTESIAN_POINT('Ctrl Pts',(-7.44282948876322,1.15322808712435,9.41561937075472));
#99559=CARTESIAN_POINT('Ctrl Pts',(-7.75660994171048,0.604759632121117,
10.2931845886062));
#99560=CARTESIAN_POINT('Ctrl Pts',(-7.11645477354922,2.32929959675149,7.64004711813815));
#99561=CARTESIAN_POINT('Ctrl Pts',(-7.29124285059876,1.7681463578603,8.53186871114499));
#99562=CARTESIAN_POINT('Ctrl Pts',(-7.57681706437927,1.21707193313286,9.40974380083951));
#99563=CARTESIAN_POINT('Ctrl Pts',(-7.88938556140438,0.668907343792867,
10.2857426732367));
#99564=CARTESIAN_POINT('Ctrl Pts',(-7.1867124928862,2.45386493727086,7.70369083485765));
#99565=CARTESIAN_POINT('Ctrl Pts',(-7.36254955939313,1.88994777765721,8.58798846945041));
#99566=CARTESIAN_POINT('Ctrl Pts',(-7.64807518901743,1.33712897273161,9.46045329326583));
#99567=CARTESIAN_POINT('Ctrl Pts',(-7.9606051534317,0.788498764169076,10.3349903948698));
#99568=CARTESIAN_POINT('Ctrl Pts',(-7.19430053092012,2.51634941530375,7.74120895321998));
#99569=CARTESIAN_POINT('Ctrl Pts',(-7.37274783895309,1.9509970957918,8.62351966308919));
#99570=CARTESIAN_POINT('Ctrl Pts',(-7.65957903289542,1.39732053099838,9.49414527429354));
#99571=CARTESIAN_POINT('Ctrl Pts',(-7.97249537063731,0.848449567099298,
10.3682028984961));
#99572=CARTESIAN_POINT('Ctrl Pts',(-7.01798682228076,1.93536441515669,8.1642169357493));
#99573=CARTESIAN_POINT('Ctrl Pts',(-7.19708258213963,1.48272786223998,8.88843542041603));
#99574=CARTESIAN_POINT('Ctrl Pts',(-7.43642528501808,1.03682530368735,9.60187951410025));
#99575=CARTESIAN_POINT('Ctrl Pts',(-7.69004994112544,0.594050075897773,
10.3103198785636));
#99576=CARTESIAN_POINT('Origin',(-7.69004994112544,0.848449567099298,10.4693195605645));
#99577=CARTESIAN_POINT('Origin',(-6.90025424549141,2.51634941530375,7.80067980343738));
#99578=CARTESIAN_POINT('Ctrl Pts',(-8.14912361676368,0.708019010352452,
10.8568386685932));
#99579=CARTESIAN_POINT('Ctrl Pts',(-8.08692216169042,0.707947174569534,
10.6858877147701));
#99580=CARTESIAN_POINT('Ctrl Pts',(-8.02503872423826,0.756217482327601,
10.5149731412681));
#99581=CARTESIAN_POINT('Ctrl Pts',(-7.97238210650343,0.848667810146629,
10.3678865203213));
#99582=CARTESIAN_POINT('Ctrl Pts',(-8.14913906922654,0.629465787637593,
10.8568651972297));
#99583=CARTESIAN_POINT('Ctrl Pts',(-8.08215444078069,0.632587778955616,
10.6730731227012));
#99584=CARTESIAN_POINT('Ctrl Pts',(-8.01637706856275,0.687463302222793,
10.4908448248287));
#99585=CARTESIAN_POINT('Ctrl Pts',(-7.96048761218811,0.788731610271473,
10.33464988296));
#99586=CARTESIAN_POINT('Ctrl Pts',(-8.08808615036661,0.472961311892115,
10.8791433605059));
#99587=CARTESIAN_POINT('Ctrl Pts',(-8.01711568751622,0.482182663833384,
10.6678349016059));
#99588=CARTESIAN_POINT('Ctrl Pts',(-7.9476905506784,0.5504216418572,10.4612353255527));
#99589=CARTESIAN_POINT('Ctrl Pts',(-7.88930781715051,0.669130461784486,
10.285312321885));
#99590=CARTESIAN_POINT('Ctrl Pts',(-7.941018055592,0.407988882551094,10.9326817955773));
#99591=CARTESIAN_POINT('Ctrl Pts',(-7.87574497017693,0.412984275736558,
10.7069427306826));
#99592=CARTESIAN_POINT('Ctrl Pts',(-7.8112653635522,0.480889739048908,10.4838995104293));
#99593=CARTESIAN_POINT('Ctrl Pts',(-7.75648913737935,0.605033293429943,
10.2927630564964));
#99594=CARTESIAN_POINT('Ctrl Pts',(-7.86720541257699,0.408000103793674,
10.9595386471957));
#99595=CARTESIAN_POINT('Ctrl Pts',(-7.80491620373291,0.407905964356341,
10.7327647510929));
#99596=CARTESIAN_POINT('Ctrl Pts',(-7.74283997308907,0.471850558728987,
10.5056555873962));
#99597=CARTESIAN_POINT('Ctrl Pts',(-7.68993326017625,0.59432004195879,10.3098881354258));
#99598=CARTESIAN_POINT('Ctrl Pts',(-7.19438354265706,2.51611178510568,7.7416193574549));
#99599=CARTESIAN_POINT('Ctrl Pts',(-7.1469608093483,2.66643382276422,7.50719050743819));
#99600=CARTESIAN_POINT('Ctrl Pts',(-7.09936908781228,2.74811551919956,7.23155382342925));
#99601=CARTESIAN_POINT('Ctrl Pts',(-7.06362916697013,2.74802300906478,6.95414127896222));
#99602=CARTESIAN_POINT('Ctrl Pts',(-7.18969017835153,2.47747072284855,7.71840107167769));
#99603=CARTESIAN_POINT('Ctrl Pts',(-7.14400277235099,2.62236748381509,7.49012436326975));
#99604=CARTESIAN_POINT('Ctrl Pts',(-7.09821965127153,2.70026704502063,7.22262797400058));
#99605=CARTESIAN_POINT('Ctrl Pts',(-7.06363490740302,2.69944028986365,6.95415602179916));
#99606=CARTESIAN_POINT('Ctrl Pts',(-7.15489990897137,2.38727021999166,7.66902358769571));
#99607=CARTESIAN_POINT('Ctrl Pts',(-7.11175827397647,2.5194913354541,7.45491010747078));
#99608=CARTESIAN_POINT('Ctrl Pts',(-7.06872790702496,2.58856514291498,7.20598605294427));
#99609=CARTESIAN_POINT('Ctrl Pts',(-7.03586871828815,2.58601736775003,6.95776948019315));
#99610=CARTESIAN_POINT('Ctrl Pts',(-7.07234001721701,2.31860209564756,7.64277634582264));
#99611=CARTESIAN_POINT('Ctrl Pts',(-7.02813588215008,2.44235324221132,7.43966879028346));
#99612=CARTESIAN_POINT('Ctrl Pts',(-6.98392692928295,2.50655355403575,7.20376129641736));
#99613=CARTESIAN_POINT('Ctrl Pts',(-6.95031555185623,2.50367339927263,6.96881823558593));
#99614=CARTESIAN_POINT('Ctrl Pts',(-7.0176774905481,2.29330136612037,7.63800974414729));
#99615=CARTESIAN_POINT('Ctrl Pts',(-6.97218688036359,2.4148874823992,7.4391751906301));
#99616=CARTESIAN_POINT('Ctrl Pts',(-6.92665536682843,2.47850902575575,7.20761906768879));
#99617=CARTESIAN_POINT('Ctrl Pts',(-6.89212767908127,2.47624041956808,6.97632364997799));
#99618=CARTESIAN_POINT('Origin',(-6.76615104985863,2.748,6.99296141887254));
#99619=CARTESIAN_POINT('Ctrl Pts',(-6.97130347175849,2.58761550236908,6.53202630652976));
#99620=CARTESIAN_POINT('Ctrl Pts',(-6.98374576415926,2.58761550236908,6.6750941373724));
#99621=CARTESIAN_POINT('Ctrl Pts',(-6.99922349531613,2.58761550236907,6.81797069470162));
#99622=CARTESIAN_POINT('Ctrl Pts',(-7.0176,2.58761550236908,6.96055403711345));
#99623=CARTESIAN_POINT('Ctrl Pts',(-7.00134514825147,2.63528330527356,6.52941364845747));
#99624=CARTESIAN_POINT('Ctrl Pts',(-7.01375047339156,2.63528330527356,6.67205641086196));
#99625=CARTESIAN_POINT('Ctrl Pts',(-7.02918337436707,2.63528330527356,6.81452097176152));
#99626=CARTESIAN_POINT('Ctrl Pts',(-7.04750769996096,2.63528330527356,6.9566994564933));
#99627=CARTESIAN_POINT('Ctrl Pts',(-7.0176,2.69159478975793,6.52799999999999));
#99628=CARTESIAN_POINT('Ctrl Pts',(-7.02998537672299,2.69159478975793,6.6704133853193));
#99629=CARTESIAN_POINT('Ctrl Pts',(-7.04539389161687,2.69159478975793,6.81265381880387));
#99630=CARTESIAN_POINT('Ctrl Pts',(-7.06369006012712,2.69159478975793,6.95461383265843));
#99631=CARTESIAN_POINT('Ctrl Pts',(-7.0176,2.748,6.52799999999999));
#99632=CARTESIAN_POINT('Ctrl Pts',(-7.02998548375468,2.748,6.67041461602438));
#99633=CARTESIAN_POINT('Ctrl Pts',(-7.04539374054221,2.748,6.8126526466152));
#99634=CARTESIAN_POINT('Ctrl Pts',(-7.06369006012712,2.748,6.95461383265843));
#99635=CARTESIAN_POINT('Origin',(0.,1.224,6.99296141887254));
#99636=CARTESIAN_POINT('',(0.,2.26194992410223,7.64168012143644));
#99637=CARTESIAN_POINT('',(0.,2.448,6.99296141887254));
#99638=CARTESIAN_POINT('Origin',(0.,2.448,7.344));
#99639=CARTESIAN_POINT('',(-2.87791997799628E-16,2.448,-9.694));
#99640=CARTESIAN_POINT('Origin',(0.,2.448,-7.344));
#99641=CARTESIAN_POINT('',(-2.87791997799628E-16,2.448,-17.854));
#99642=CARTESIAN_POINT('Origin',(0.,2.448,-15.504));
#99643=CARTESIAN_POINT('Origin',(6.528,0.708,42.432));
#99644=CARTESIAN_POINT('',(6.528,0.708,41.132));
#99645=CARTESIAN_POINT('Origin',(6.528,0.708,40.832));
#99646=CARTESIAN_POINT('',(5.228,0.708,42.432));
#99647=CARTESIAN_POINT('Origin',(6.528,0.708,42.432));
#99648=CARTESIAN_POINT('Origin',(6.528,0.708,42.432));
#99649=CARTESIAN_POINT('Origin',(6.528,-4.08,42.432));
#99650=CARTESIAN_POINT('',(5.228,0.924,42.432));
#99651=CARTESIAN_POINT('',(5.228,-4.08,42.432));
#99652=CARTESIAN_POINT('',(6.528,0.924,43.732));
#99653=CARTESIAN_POINT('Origin',(6.528,0.924,42.432));
#99654=CARTESIAN_POINT('Origin',(6.528,0.924,42.432));
#99655=CARTESIAN_POINT('Origin',(6.528,0.924,42.432));
#99656=CARTESIAN_POINT('Origin',(6.528,0.924,44.032));
#99657=CARTESIAN_POINT('Origin',(0.,2.748,-7.344));
#99658=CARTESIAN_POINT('',(-2.51052593825207E-16,2.748,-9.394));
#99659=CARTESIAN_POINT('Origin',(-2.87791997799628E-16,2.748,-9.694));
#99660=CARTESIAN_POINT('',(-2.05,2.748,-7.344));
#99661=CARTESIAN_POINT('Origin',(0.,2.748,-7.344));
#99662=CARTESIAN_POINT('Origin',(0.,2.748,-7.344));
#99663=CARTESIAN_POINT('Origin',(0.,-4.08,-7.344));
#99664=CARTESIAN_POINT('',(-2.05,2.964,-7.344));
#99665=CARTESIAN_POINT('',(-2.05,-4.08,-7.344));
#99666=CARTESIAN_POINT('',(-2.51052593825207E-16,2.964,-5.294));
#99667=CARTESIAN_POINT('Origin',(0.,2.964,-7.344));
#99668=CARTESIAN_POINT('Origin',(0.,2.964,-7.344));
#99669=CARTESIAN_POINT('Origin',(0.,2.964,-7.344));
#99670=CARTESIAN_POINT('',(-2.87791997799628E-16,3.264,-4.994));
#99671=CARTESIAN_POINT('Origin',(0.,3.264,-7.344));
#99672=CARTESIAN_POINT('Origin',(-2.87791997799628E-16,2.964,-4.994));
#99673=CARTESIAN_POINT('Origin',(0.,3.264,-24.48));
#99674=CARTESIAN_POINT('',(0.,3.264,7.31936141887254));
#99675=CARTESIAN_POINT('',(-2.87791997799628E-16,3.264,-13.154));
#99676=CARTESIAN_POINT('Origin',(0.,3.264,-15.504));
#99677=CARTESIAN_POINT('Origin',(-6.528,0.708,42.432));
#99678=CARTESIAN_POINT('',(-6.528,0.708,41.132));
#99679=CARTESIAN_POINT('Origin',(-6.528,0.708,40.832));
#99680=CARTESIAN_POINT('',(-7.828,0.708,42.432));
#99681=CARTESIAN_POINT('Origin',(-6.528,0.708,42.432));
#99682=CARTESIAN_POINT('Origin',(-6.528,0.708,42.432));
#99683=CARTESIAN_POINT('Origin',(-6.528,-4.08,42.432));
#99684=CARTESIAN_POINT('',(-7.828,0.924,42.432));
#99685=CARTESIAN_POINT('',(-7.828,-4.08,42.432));
#99686=CARTESIAN_POINT('',(-6.528,0.924,43.732));
#99687=CARTESIAN_POINT('Origin',(-6.528,0.924,42.432));
#99688=CARTESIAN_POINT('Origin',(-6.528,0.924,42.432));
#99689=CARTESIAN_POINT('Origin',(-6.528,0.924,42.432));
#99690=CARTESIAN_POINT('Origin',(-6.528,0.924,44.032));
#99691=CARTESIAN_POINT('Origin',(0.,2.748,-15.504));
#99692=CARTESIAN_POINT('',(-2.51052593825207E-16,2.748,-17.554));
#99693=CARTESIAN_POINT('Origin',(-2.87791997799628E-16,2.748,-17.854));
#99694=CARTESIAN_POINT('',(-2.05,2.748,-15.504));
#99695=CARTESIAN_POINT('Origin',(0.,2.748,-15.504));
#99696=CARTESIAN_POINT('Origin',(0.,2.748,-15.504));
#99697=CARTESIAN_POINT('Origin',(0.,-4.08,-15.504));
#99698=CARTESIAN_POINT('',(-2.05,2.964,-15.504));
#99699=CARTESIAN_POINT('',(-2.05,-4.08,-15.504));
#99700=CARTESIAN_POINT('',(-2.51052593825207E-16,2.964,-13.454));
#99701=CARTESIAN_POINT('Origin',(0.,2.964,-15.504));
#99702=CARTESIAN_POINT('Origin',(0.,2.964,-15.504));
#99703=CARTESIAN_POINT('Origin',(0.,2.964,-15.504));
#99704=CARTESIAN_POINT('Origin',(-2.87791997799628E-16,2.964,-13.154));
#99705=CARTESIAN_POINT('Origin',(0.,0.408,10.608));
#99706=CARTESIAN_POINT('Origin',(0.,2.04,7.31936141887254));
#99707=CARTESIAN_POINT('',(0.,3.07794992410223,7.96808012143643));
#99708=CARTESIAN_POINT('Origin',(0.,2.448,11.2854385811275));
#99709=CARTESIAN_POINT('',(0.,1.41005007589777,10.6367198785636));
#99710=CARTESIAN_POINT('Origin',(0.,3.264,7.6704));
#100002=UNCERTAINTY_MEASURE_WITH_UNIT(LENGTH_MEASURE(0.01),#100032,
'DISTANCE_ACCURACY_VALUE',
'Maximum model space distance between geometric entities at asserted c
onnectivities');
#100011=UNCERTAINTY_MEASURE_WITH_UNIT(LENGTH_MEASURE(0.01),#100032,
'DISTANCE_ACCURACY_VALUE',
'Maximum model space distance between geometric entities at asserted c
onnectivities');
#100022=(
GEOMETRIC_REPRESENTATION_CONTEXT(3)
GLOBAL_UNCERTAINTY_ASSIGNED_CONTEXT((#100002))
GLOBAL_UNIT_ASSIGNED_CONTEXT((#100032,#100034,#100035))
REPRESENTATION_CONTEXT('','3D')
);
#100031=(
GEOMETRIC_REPRESENTATION_CONTEXT(3)
GLOBAL_UNCERTAINTY_ASSIGNED_CONTEXT((#100011))
GLOBAL_UNIT_ASSIGNED_CONTEXT((#100032,#100034,#100035))
REPRESENTATION_CONTEXT('','3D')
);
#100032=(
LENGTH_UNIT()
NAMED_UNIT(*)
SI_UNIT(.MILLI.,.METRE.)
);
#100034=(
NAMED_UNIT(*)
PLANE_ANGLE_UNIT()
SI_UNIT($,.RADIAN.)
);
#100035=(
NAMED_UNIT(*)
SI_UNIT($,.STERADIAN.)
SOLID_ANGLE_UNIT()
);
#100046=SHAPE_DEFINITION_REPRESENTATION(#100065,#100110);
#100065=PRODUCT_DEFINITION_SHAPE('',$,#100130);
#100110=SHAPE_REPRESENTATION('',(#22218),#100022);
#100119=PRODUCT_DEFINITION_CONTEXT('part definition',#100178,'design');
#100130=PRODUCT_DEFINITION('2026-10-12-11-55-30-112',
'18_Coupling_Cover_Leaf_Plate',#100149,#100119);
#100149=PRODUCT_DEFINITION_FORMATION('',$,#100190);
#100178=APPLICATION_CONTEXT(
'Core Data for Automotive Mechanical Design Process');
#100179=PRODUCT_CONTEXT('part definition',#100178,'mechanical');
#100190=PRODUCT('2026-10-12-11-55-30-112',
'18_Coupling_Cover_Leaf_Plate',$,(#100179));
#100200=PRESENTATION_STYLE_ASSIGNMENT((#100206));
#100206=SURFACE_STYLE_USAGE(.BOTH.,#100212);
#100212=SURFACE_SIDE_STYLE('',(#100218));
#100218=SURFACE_STYLE_FILL_AREA(#100224);
#100224=FILL_AREA_STYLE('Opaque(227,224,212)',(#100230));
#100230=FILL_AREA_STYLE_COLOUR('Opaque(227,224,212)',#100236);
#100236=COLOUR_RGB('Opaque(227,224,212)',0.890196078431372,0.87843137254902,
0.831372549019608);
ENDSEC;
END-ISO-10303-21;
